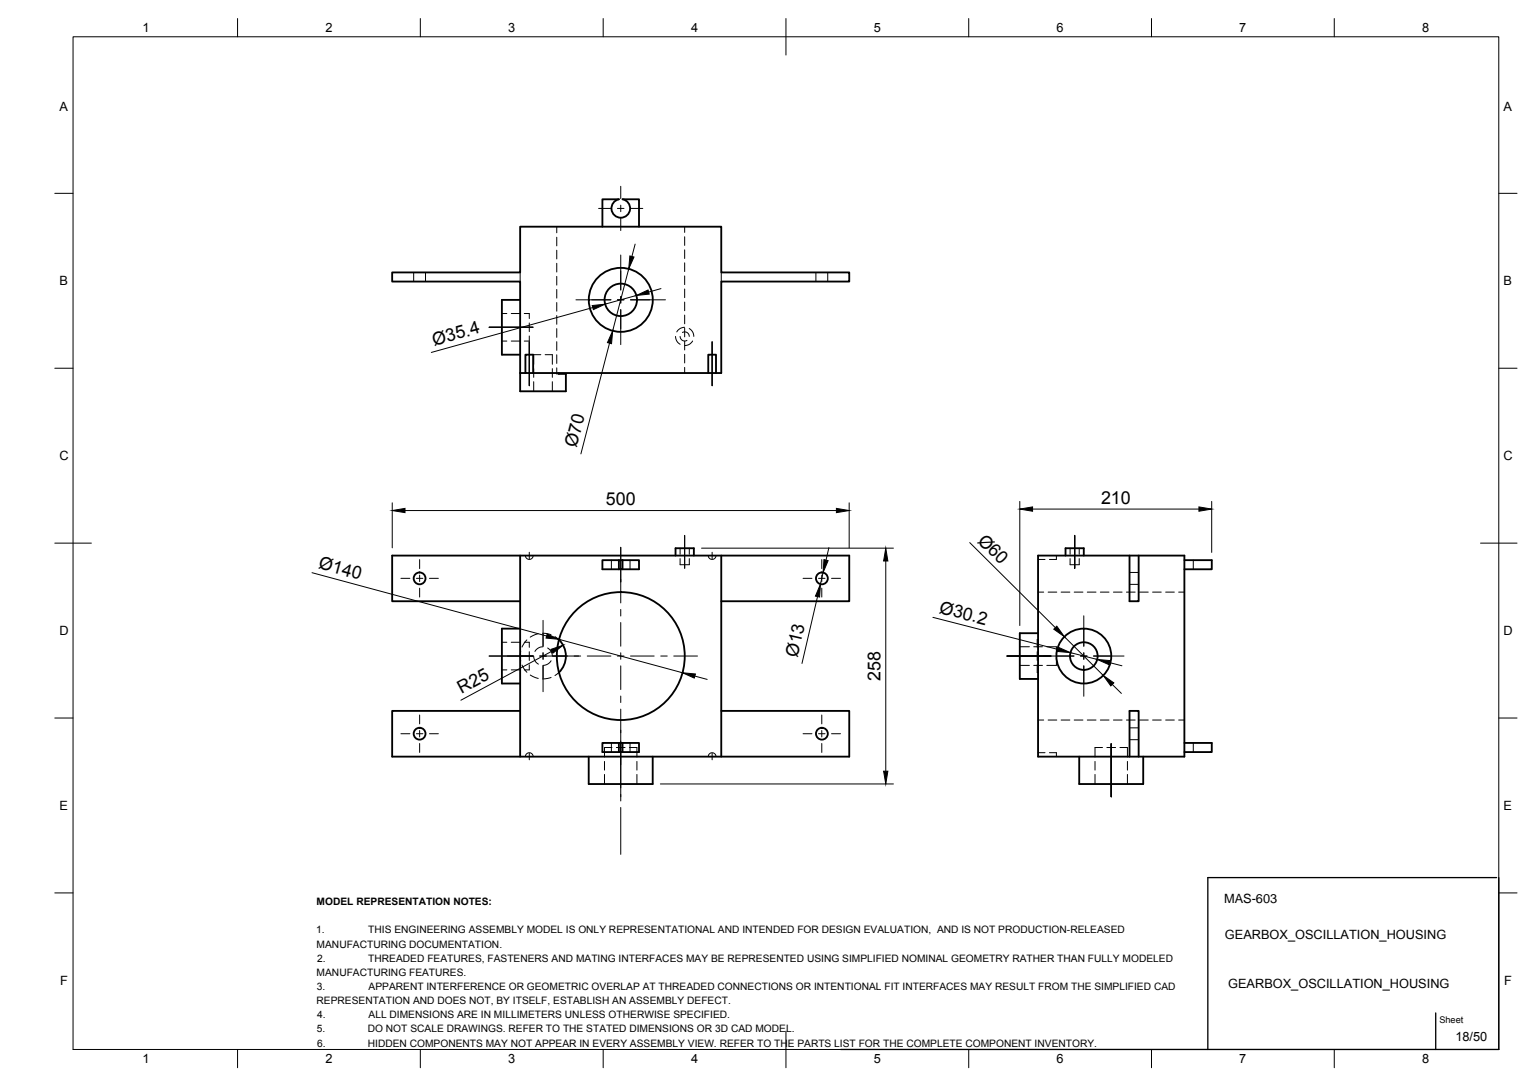
ISO-10303-21;
HEADER;
FILE_DESCRIPTION((''),'2;1');
FILE_NAME('GEARBOX_OSCILLATION_HOUSING.step','2026-10-01T22:06:14-07:00',(''),(''),'','','');
FILE_SCHEMA (('AUTOMOTIVE_DESIGN { 1 0 10303 214 3 1 1 }'));
ENDSEC;
DATA;
#10=MECHANICAL_DESIGN_GEOMETRIC_PRESENTATION_REPRESENTATION('',(#990),#50440);
#900=SHAPE_REPRESENTATION_RELATIONSHIP('SRR','None',#50632,#945) ;
#945=ADVANCED_BREP_SHAPE_REPRESENTATION('',(#1045),#50401) ;
#990=STYLED_ITEM('',(#50886),#1045) ;
#1045=MANIFOLD_SOLID_BREP('GEARBOX_OSCILLATION_HOUSING',#28657) ;
#1276=FACE_BOUND('',#4753,.T.) ;
#1277=FACE_BOUND('',#4757,.T.) ;
#1278=FACE_BOUND('',#4764,.T.) ;
#1279=FACE_BOUND('',#4785,.T.) ;
#1280=FACE_BOUND('',#4790,.T.) ;
#1281=FACE_BOUND('',#4795,.T.) ;
#1282=FACE_BOUND('',#4797,.T.) ;
#1283=FACE_BOUND('',#4799,.T.) ;
#1284=FACE_BOUND('',#4803,.T.) ;
#1285=FACE_BOUND('',#4805,.T.) ;
#1286=FACE_BOUND('',#4807,.T.) ;
#1287=FACE_BOUND('',#4811,.T.) ;
#1288=FACE_BOUND('',#4813,.T.) ;
#1289=FACE_BOUND('',#4817,.T.) ;
#1290=FACE_BOUND('',#4819,.T.) ;
#1291=FACE_BOUND('',#4824,.T.) ;
#1292=FACE_BOUND('',#4825,.T.) ;
#1293=FACE_BOUND('',#4826,.T.) ;
#1932=PLANE('',#30300) ;
#1933=PLANE('',#30301) ;
#1934=PLANE('',#30310) ;
#1935=PLANE('',#30313) ;
#1936=PLANE('',#30315) ;
#1937=PLANE('',#30318) ;
#1938=PLANE('',#30320) ;
#1939=PLANE('',#30326) ;
#1940=PLANE('',#30329) ;
#1941=PLANE('',#30336) ;
#1942=PLANE('',#30337) ;
#1943=PLANE('',#30338) ;
#1944=PLANE('',#30339) ;
#1945=PLANE('',#30340) ;
#1946=PLANE('',#30341) ;
#1947=PLANE('',#30342) ;
#1948=PLANE('',#30343) ;
#1949=PLANE('',#30344) ;
#1950=PLANE('',#30345) ;
#1951=PLANE('',#30346) ;
#1952=PLANE('',#30347) ;
#1953=PLANE('',#30348) ;
#1954=PLANE('',#30358) ;
#1955=PLANE('',#30359) ;
#1956=PLANE('',#30363) ;
#1957=PLANE('',#30367) ;
#1958=PLANE('',#30371) ;
#1959=PLANE('',#30374) ;
#1960=PLANE('',#30375) ;
#1961=PLANE('',#30376) ;
#1962=PLANE('',#30377) ;
#1963=PLANE('',#30378) ;
#1964=PLANE('',#30379) ;
#1965=PLANE('',#30380) ;
#1966=PLANE('',#30381) ;
#1967=PLANE('',#30382) ;
#1968=PLANE('',#30383) ;
#1969=PLANE('',#30384) ;
#1970=PLANE('',#30385) ;
#1971=PLANE('',#30386) ;
#1972=PLANE('',#30387) ;
#1973=PLANE('',#30388) ;
#1974=PLANE('',#30389) ;
#1975=PLANE('',#30390) ;
#1976=PLANE('',#30391) ;
#1977=PLANE('',#30392) ;
#1978=PLANE('',#30393) ;
#3025=FACE_OUTER_BOUND('',#4743,.T.) ;
#3026=FACE_OUTER_BOUND('',#4744,.T.) ;
#3027=FACE_OUTER_BOUND('',#4745,.T.) ;
#3028=FACE_OUTER_BOUND('',#4746,.T.) ;
#3029=FACE_OUTER_BOUND('',#4747,.T.) ;
#3030=FACE_OUTER_BOUND('',#4748,.T.) ;
#3031=FACE_OUTER_BOUND('',#4749,.T.) ;
#3032=FACE_OUTER_BOUND('',#4750,.T.) ;
#3033=FACE_OUTER_BOUND('',#4751,.T.) ;
#3034=FACE_OUTER_BOUND('',#4752,.T.) ;
#3035=FACE_OUTER_BOUND('',#4754,.T.) ;
#3036=FACE_OUTER_BOUND('',#4755,.T.) ;
#3037=FACE_OUTER_BOUND('',#4756,.T.) ;
#3038=FACE_OUTER_BOUND('',#4758,.T.) ;
#3039=FACE_OUTER_BOUND('',#4759,.T.) ;
#3040=FACE_OUTER_BOUND('',#4760,.T.) ;
#3041=FACE_OUTER_BOUND('',#4761,.T.) ;
#3042=FACE_OUTER_BOUND('',#4762,.T.) ;
#3043=FACE_OUTER_BOUND('',#4763,.T.) ;
#3044=FACE_OUTER_BOUND('',#4765,.T.) ;
#3045=FACE_OUTER_BOUND('',#4766,.T.) ;
#3046=FACE_OUTER_BOUND('',#4767,.T.) ;
#3047=FACE_OUTER_BOUND('',#4768,.T.) ;
#3048=FACE_OUTER_BOUND('',#4769,.T.) ;
#3049=FACE_OUTER_BOUND('',#4770,.T.) ;
#3050=FACE_OUTER_BOUND('',#4771,.T.) ;
#3051=FACE_OUTER_BOUND('',#4772,.T.) ;
#3052=FACE_OUTER_BOUND('',#4773,.T.) ;
#3053=FACE_OUTER_BOUND('',#4774,.T.) ;
#3054=FACE_OUTER_BOUND('',#4775,.T.) ;
#3055=FACE_OUTER_BOUND('',#4776,.T.) ;
#3056=FACE_OUTER_BOUND('',#4777,.T.) ;
#3057=FACE_OUTER_BOUND('',#4778,.T.) ;
#3058=FACE_OUTER_BOUND('',#4779,.T.) ;
#3059=FACE_OUTER_BOUND('',#4780,.T.) ;
#3060=FACE_OUTER_BOUND('',#4781,.T.) ;
#3061=FACE_OUTER_BOUND('',#4782,.T.) ;
#3062=FACE_OUTER_BOUND('',#4783,.T.) ;
#3063=FACE_OUTER_BOUND('',#4784,.T.) ;
#3064=FACE_OUTER_BOUND('',#4786,.T.) ;
#3065=FACE_OUTER_BOUND('',#4787,.T.) ;
#3066=FACE_OUTER_BOUND('',#4788,.T.) ;
#3067=FACE_OUTER_BOUND('',#4789,.T.) ;
#3068=FACE_OUTER_BOUND('',#4791,.T.) ;
#3069=FACE_OUTER_BOUND('',#4792,.T.) ;
#3070=FACE_OUTER_BOUND('',#4793,.T.) ;
#3071=FACE_OUTER_BOUND('',#4794,.T.) ;
#3072=FACE_OUTER_BOUND('',#4796,.T.) ;
#3073=FACE_OUTER_BOUND('',#4798,.T.) ;
#3074=FACE_OUTER_BOUND('',#4800,.T.) ;
#3075=FACE_OUTER_BOUND('',#4801,.T.) ;
#3076=FACE_OUTER_BOUND('',#4802,.T.) ;
#3077=FACE_OUTER_BOUND('',#4804,.T.) ;
#3078=FACE_OUTER_BOUND('',#4806,.T.) ;
#3079=FACE_OUTER_BOUND('',#4808,.T.) ;
#3080=FACE_OUTER_BOUND('',#4809,.T.) ;
#3081=FACE_OUTER_BOUND('',#4810,.T.) ;
#3082=FACE_OUTER_BOUND('',#4812,.T.) ;
#3083=FACE_OUTER_BOUND('',#4814,.T.) ;
#3084=FACE_OUTER_BOUND('',#4815,.T.) ;
#3085=FACE_OUTER_BOUND('',#4816,.T.) ;
#3086=FACE_OUTER_BOUND('',#4818,.T.) ;
#3087=FACE_OUTER_BOUND('',#4820,.T.) ;
#3088=FACE_OUTER_BOUND('',#4821,.T.) ;
#3089=FACE_OUTER_BOUND('',#4822,.T.) ;
#3090=FACE_OUTER_BOUND('',#4823,.T.) ;
#4743=EDGE_LOOP('',(#22155,#22156,#22157,#22158)) ;
#4744=EDGE_LOOP('',(#22159,#22160,#22161,#22162)) ;
#4745=EDGE_LOOP('',(#22163,#22164,#22165,#22166)) ;
#4746=EDGE_LOOP('',(#22167,#22168,#22169,#22170)) ;
#4747=EDGE_LOOP('',(#22171,#22172,#22173,#22174)) ;
#4748=EDGE_LOOP('',(#22175,#22176)) ;
#4749=EDGE_LOOP('',(#22177,#22178,#22179,#22180,#22181,#22182,#22183,#22184,
#22185,#22186,#22187,#22188,#22189,#22190,#22191,#22192,#22193,#22194)) ;
#4750=EDGE_LOOP('',(#22195,#22196)) ;
#4751=EDGE_LOOP('',(#22197,#22198,#22199,#22200)) ;
#4752=EDGE_LOOP('',(#22201,#22202,#22203,#22204,#22205,#22206,#22207,#22208,
#22209,#22210,#22211,#22212,#22213,#22214,#22215,#22216,#22217,#22218,#22219,
#22220)) ;
#4753=EDGE_LOOP('',(#22221)) ;
#4754=EDGE_LOOP('',(#22222,#22223)) ;
#4755=EDGE_LOOP('',(#22224,#22225,#22226,#22227)) ;
#4756=EDGE_LOOP('',(#22228,#22229,#22230,#22231,#22232,#22233,#22234,#22235,
#22236,#22237,#22238,#22239,#22240,#22241,#22242,#22243,#22244,#22245,#22246,
#22247)) ;
#4757=EDGE_LOOP('',(#22248)) ;
#4758=EDGE_LOOP('',(#22249,#22250)) ;
#4759=EDGE_LOOP('',(#22251,#22252,#22253,#22254)) ;
#4760=EDGE_LOOP('',(#22255,#22256,#22257,#22258)) ;
#4761=EDGE_LOOP('',(#22259)) ;
#4762=EDGE_LOOP('',(#22260,#22261,#22262,#22263)) ;
#4763=EDGE_LOOP('',(#22264)) ;
#4764=EDGE_LOOP('',(#22265)) ;
#4765=EDGE_LOOP('',(#22266,#22267,#22268,#22269)) ;
#4766=EDGE_LOOP('',(#22270,#22271,#22272,#22273)) ;
#4767=EDGE_LOOP('',(#22274,#22275,#22276,#22277,#22278,#22279)) ;
#4768=EDGE_LOOP('',(#22280,#22281,#22282,#22283)) ;
#4769=EDGE_LOOP('',(#22284,#22285,#22286,#22287)) ;
#4770=EDGE_LOOP('',(#22288,#22289,#22290,#22291,#22292,#22293)) ;
#4771=EDGE_LOOP('',(#22294,#22295,#22296,#22297)) ;
#4772=EDGE_LOOP('',(#22298,#22299,#22300,#22301)) ;
#4773=EDGE_LOOP('',(#22302,#22303,#22304,#22305)) ;
#4774=EDGE_LOOP('',(#22306,#22307,#22308,#22309)) ;
#4775=EDGE_LOOP('',(#22310,#22311,#22312,#22313,#22314,#22315)) ;
#4776=EDGE_LOOP('',(#22316,#22317,#22318,#22319)) ;
#4777=EDGE_LOOP('',(#22320,#22321,#22322,#22323)) ;
#4778=EDGE_LOOP('',(#22324,#22325,#22326,#22327,#22328,#22329)) ;
#4779=EDGE_LOOP('',(#22330,#22331)) ;
#4780=EDGE_LOOP('',(#22332,#22333,#22334,#22335,#22336,#22337,#22338,#22339)) ;
#4781=EDGE_LOOP('',(#22340,#22341,#22342,#22343,#22344,#22345,#22346,#22347,
#22348)) ;
#4782=EDGE_LOOP('',(#22349,#22350,#22351,#22352)) ;
#4783=EDGE_LOOP('',(#22353)) ;
#4784=EDGE_LOOP('',(#22354)) ;
#4785=EDGE_LOOP('',(#22355)) ;
#4786=EDGE_LOOP('',(#22356,#22357,#22358,#22359)) ;
#4787=EDGE_LOOP('',(#22360)) ;
#4788=EDGE_LOOP('',(#22361,#22362,#22363,#22364)) ;
#4789=EDGE_LOOP('',(#22365)) ;
#4790=EDGE_LOOP('',(#22366)) ;
#4791=EDGE_LOOP('',(#22367,#22368,#22369,#22370)) ;
#4792=EDGE_LOOP('',(#22371)) ;
#4793=EDGE_LOOP('',(#22372,#22373,#22374,#22375)) ;
#4794=EDGE_LOOP('',(#22376)) ;
#4795=EDGE_LOOP('',(#22377)) ;
#4796=EDGE_LOOP('',(#22378,#22379,#22380,#22381)) ;
#4797=EDGE_LOOP('',(#22382)) ;
#4798=EDGE_LOOP('',(#22383,#22384,#22385,#22386)) ;
#4799=EDGE_LOOP('',(#22387)) ;
#4800=EDGE_LOOP('',(#22388,#22389,#22390,#22391)) ;
#4801=EDGE_LOOP('',(#22392,#22393,#22394,#22395)) ;
#4802=EDGE_LOOP('',(#22396,#22397,#22398,#22399,#22400,#22401,#22402,#22403,
#22404,#22405,#22406,#22407,#22408)) ;
#4803=EDGE_LOOP('',(#22409)) ;
#4804=EDGE_LOOP('',(#22410,#22411,#22412,#22413)) ;
#4805=EDGE_LOOP('',(#22414)) ;
#4806=EDGE_LOOP('',(#22415,#22416,#22417,#22418)) ;
#4807=EDGE_LOOP('',(#22419)) ;
#4808=EDGE_LOOP('',(#22420,#22421,#22422,#22423)) ;
#4809=EDGE_LOOP('',(#22424,#22425,#22426,#22427)) ;
#4810=EDGE_LOOP('',(#22428,#22429,#22430,#22431)) ;
#4811=EDGE_LOOP('',(#22432)) ;
#4812=EDGE_LOOP('',(#22433,#22434,#22435,#22436)) ;
#4813=EDGE_LOOP('',(#22437)) ;
#4814=EDGE_LOOP('',(#22438,#22439,#22440,#22441)) ;
#4815=EDGE_LOOP('',(#22442,#22443,#22444,#22445)) ;
#4816=EDGE_LOOP('',(#22446,#22447,#22448,#22449)) ;
#4817=EDGE_LOOP('',(#22450)) ;
#4818=EDGE_LOOP('',(#22451,#22452,#22453,#22454)) ;
#4819=EDGE_LOOP('',(#22455)) ;
#4820=EDGE_LOOP('',(#22456,#22457,#22458,#22459)) ;
#4821=EDGE_LOOP('',(#22460,#22461,#22462,#22463)) ;
#4822=EDGE_LOOP('',(#22464,#22465,#22466,#22467,#22468,#22469,#22470,#22471,
#22472,#22473,#22474,#22475)) ;
#4823=EDGE_LOOP('',(#22476,#22477,#22478,#22479)) ;
#4824=EDGE_LOOP('',(#22480,#22481,#22482,#22483)) ;
#4825=EDGE_LOOP('',(#22484,#22485,#22486,#22487)) ;
#4826=EDGE_LOOP('',(#22488)) ;
#7141=LINE('',#45071,#9613) ;
#7142=LINE('',#45077,#9614) ;
#7143=LINE('',#45083,#9615) ;
#7144=LINE('',#45089,#9616) ;
#7145=LINE('',#45094,#9617) ;
#7146=LINE('',#45098,#9618) ;
#7147=LINE('',#45101,#9619) ;
#7148=LINE('',#45104,#9620) ;
#7149=LINE('',#45106,#9621) ;
#7150=LINE('',#45117,#9622) ;
#7151=LINE('',#45119,#9623) ;
#7152=LINE('',#45123,#9624) ;
#7153=LINE('',#45127,#9625) ;
#7154=LINE('',#45129,#9626) ;
#7155=LINE('',#45131,#9627) ;
#7156=LINE('',#45134,#9628) ;
#7157=LINE('',#45138,#9629) ;
#7158=LINE('',#45141,#9630) ;
#7159=LINE('',#45142,#9631) ;
#7160=LINE('',#45145,#9632) ;
#7161=LINE('',#45147,#9633) ;
#7162=LINE('',#45149,#9634) ;
#7163=LINE('',#45151,#9635) ;
#7164=LINE('',#45153,#9636) ;
#7165=LINE('',#45155,#9637) ;
#7166=LINE('',#45157,#9638) ;
#7167=LINE('',#45159,#9639) ;
#7168=LINE('',#45161,#9640) ;
#7169=LINE('',#45163,#9641) ;
#7170=LINE('',#45164,#9642) ;
#7171=LINE('',#45170,#9643) ;
#7172=LINE('',#45173,#9644) ;
#7173=LINE('',#45174,#9645) ;
#7174=LINE('',#45177,#9646) ;
#7175=LINE('',#45179,#9647) ;
#7176=LINE('',#45181,#9648) ;
#7177=LINE('',#45183,#9649) ;
#7178=LINE('',#45185,#9650) ;
#7179=LINE('',#45187,#9651) ;
#7180=LINE('',#45189,#9652) ;
#7181=LINE('',#45191,#9653) ;
#7182=LINE('',#45193,#9654) ;
#7183=LINE('',#45195,#9655) ;
#7184=LINE('',#45196,#9656) ;
#7185=LINE('',#45198,#9657) ;
#7186=LINE('',#45200,#9658) ;
#7187=LINE('',#45201,#9659) ;
#7188=LINE('',#45211,#9660) ;
#7189=LINE('',#45217,#9661) ;
#7190=LINE('',#45222,#9662) ;
#7191=LINE('',#45226,#9663) ;
#7192=LINE('',#45231,#9664) ;
#7193=LINE('',#45235,#9665) ;
#7194=LINE('',#45239,#9666) ;
#7195=LINE('',#45241,#9667) ;
#7196=LINE('',#45243,#9668) ;
#7197=LINE('',#45245,#9669) ;
#7198=LINE('',#45246,#9670) ;
#7199=LINE('',#45249,#9671) ;
#7200=LINE('',#45250,#9672) ;
#7201=LINE('',#45253,#9673) ;
#7202=LINE('',#45254,#9674) ;
#7203=LINE('',#45257,#9675) ;
#7204=LINE('',#45259,#9676) ;
#7205=LINE('',#45261,#9677) ;
#7206=LINE('',#45263,#9678) ;
#7207=LINE('',#45264,#9679) ;
#7208=LINE('',#45267,#9680) ;
#7209=LINE('',#45268,#9681) ;
#7210=LINE('',#45271,#9682) ;
#7211=LINE('',#45272,#9683) ;
#7212=LINE('',#45275,#9684) ;
#7213=LINE('',#45276,#9685) ;
#7214=LINE('',#45279,#9686) ;
#7215=LINE('',#45280,#9687) ;
#7216=LINE('',#45282,#9688) ;
#7217=LINE('',#45285,#9689) ;
#7218=LINE('',#45286,#9690) ;
#7219=LINE('',#45289,#9691) ;
#7220=LINE('',#45290,#9692) ;
#7221=LINE('',#45292,#9693) ;
#7222=LINE('',#45301,#9694) ;
#7223=LINE('',#45302,#9695) ;
#7224=LINE('',#45303,#9696) ;
#7225=LINE('',#45307,#9697) ;
#7226=LINE('',#45312,#9698) ;
#7227=LINE('',#45320,#9699) ;
#7228=LINE('',#45327,#9700) ;
#7229=LINE('',#45334,#9701) ;
#7230=LINE('',#45339,#9702) ;
#7231=LINE('',#45345,#9703) ;
#7232=LINE('',#45346,#9704) ;
#7233=LINE('',#45347,#9705) ;
#7234=LINE('',#45351,#9706) ;
#7235=LINE('',#45352,#9707) ;
#7236=LINE('',#45353,#9708) ;
#7237=LINE('',#45355,#9709) ;
#7238=LINE('',#45357,#9710) ;
#7239=LINE('',#45359,#9711) ;
#7240=LINE('',#45361,#9712) ;
#7241=LINE('',#45363,#9713) ;
#7242=LINE('',#45364,#9714) ;
#7243=LINE('',#45368,#9715) ;
#7244=LINE('',#45369,#9716) ;
#7245=LINE('',#45370,#9717) ;
#7246=LINE('',#45374,#9718) ;
#7247=LINE('',#45375,#9719) ;
#7248=LINE('',#45376,#9720) ;
#7249=LINE('',#45378,#9721) ;
#7250=LINE('',#45380,#9722) ;
#7251=LINE('',#45383,#9723) ;
#7252=LINE('',#45384,#9724) ;
#7253=LINE('',#45387,#9725) ;
#7254=LINE('',#45388,#9726) ;
#7255=LINE('',#45390,#9727) ;
#7256=LINE('',#45394,#9728) ;
#7257=LINE('',#45396,#9729) ;
#7258=LINE('',#45397,#9730) ;
#7259=LINE('',#45400,#9731) ;
#7260=LINE('',#45402,#9732) ;
#7261=LINE('',#45403,#9733) ;
#7262=LINE('',#45405,#9734) ;
#7263=LINE('',#45406,#9735) ;
#7264=LINE('',#45409,#9736) ;
#9613=VECTOR('',#35940,0.65) ;
#9614=VECTOR('',#35947,0.65) ;
#9615=VECTOR('',#35954,0.65) ;
#9616=VECTOR('',#35961,0.65) ;
#9617=VECTOR('',#35966,1.) ;
#9618=VECTOR('',#35969,1.) ;
#9619=VECTOR('',#35974,1.) ;
#9620=VECTOR('',#35977,1.) ;
#9621=VECTOR('',#35978,1.) ;
#9622=VECTOR('',#35989,1.) ;
#9623=VECTOR('',#35990,1.) ;
#9624=VECTOR('',#35993,1.) ;
#9625=VECTOR('',#35996,1.) ;
#9626=VECTOR('',#35997,1.) ;
#9627=VECTOR('',#35998,1.) ;
#9628=VECTOR('',#36001,1.) ;
#9629=VECTOR('',#36004,1.) ;
#9630=VECTOR('',#36009,1.) ;
#9631=VECTOR('',#36010,1.) ;
#9632=VECTOR('',#36013,1.) ;
#9633=VECTOR('',#36014,1.) ;
#9634=VECTOR('',#36015,1.) ;
#9635=VECTOR('',#36016,1.) ;
#9636=VECTOR('',#36017,1.) ;
#9637=VECTOR('',#36018,1.) ;
#9638=VECTOR('',#36019,1.) ;
#9639=VECTOR('',#36020,1.) ;
#9640=VECTOR('',#36021,1.) ;
#9641=VECTOR('',#36022,1.) ;
#9642=VECTOR('',#36023,1.) ;
#9643=VECTOR('',#36028,1.) ;
#9644=VECTOR('',#36033,1.) ;
#9645=VECTOR('',#36034,1.) ;
#9646=VECTOR('',#36037,1.) ;
#9647=VECTOR('',#36038,1.) ;
#9648=VECTOR('',#36039,1.) ;
#9649=VECTOR('',#36040,1.) ;
#9650=VECTOR('',#36041,1.) ;
#9651=VECTOR('',#36042,1.) ;
#9652=VECTOR('',#36043,1.) ;
#9653=VECTOR('',#36044,1.) ;
#9654=VECTOR('',#36045,1.) ;
#9655=VECTOR('',#36046,1.) ;
#9656=VECTOR('',#36047,1.) ;
#9657=VECTOR('',#36048,1.) ;
#9658=VECTOR('',#36049,1.) ;
#9659=VECTOR('',#36050,1.) ;
#9660=VECTOR('',#36063,0.5) ;
#9661=VECTOR('',#36072,1.) ;
#9662=VECTOR('',#36077,1.) ;
#9663=VECTOR('',#36080,1.) ;
#9664=VECTOR('',#36085,1.) ;
#9665=VECTOR('',#36088,1.) ;
#9666=VECTOR('',#36093,1.) ;
#9667=VECTOR('',#36094,1.) ;
#9668=VECTOR('',#36095,1.) ;
#9669=VECTOR('',#36096,1.) ;
#9670=VECTOR('',#36097,1.) ;
#9671=VECTOR('',#36100,1.) ;
#9672=VECTOR('',#36101,1.) ;
#9673=VECTOR('',#36104,1.) ;
#9674=VECTOR('',#36105,1.) ;
#9675=VECTOR('',#36108,1.) ;
#9676=VECTOR('',#36109,1.) ;
#9677=VECTOR('',#36110,1.) ;
#9678=VECTOR('',#36111,1.) ;
#9679=VECTOR('',#36112,1.) ;
#9680=VECTOR('',#36115,1.) ;
#9681=VECTOR('',#36116,1.) ;
#9682=VECTOR('',#36119,1.) ;
#9683=VECTOR('',#36120,1.) ;
#9684=VECTOR('',#36123,1.) ;
#9685=VECTOR('',#36124,1.) ;
#9686=VECTOR('',#36127,1.) ;
#9687=VECTOR('',#36128,1.) ;
#9688=VECTOR('',#36131,1.) ;
#9689=VECTOR('',#36134,1.) ;
#9690=VECTOR('',#36135,1.) ;
#9691=VECTOR('',#36138,1.) ;
#9692=VECTOR('',#36139,1.) ;
#9693=VECTOR('',#36142,1.) ;
#9694=VECTOR('',#36153,7.) ;
#9695=VECTOR('',#36154,1.) ;
#9696=VECTOR('',#36155,1.) ;
#9697=VECTOR('',#36160,2.5) ;
#9698=VECTOR('',#36165,1.02) ;
#9699=VECTOR('',#36176,1.51) ;
#9700=VECTOR('',#36185,3.) ;
#9701=VECTOR('',#36194,1.77) ;
#9702=VECTOR('',#36201,3.5) ;
#9703=VECTOR('',#36208,1.) ;
#9704=VECTOR('',#36209,1.) ;
#9705=VECTOR('',#36210,1.) ;
#9706=VECTOR('',#36213,1.) ;
#9707=VECTOR('',#36214,1.) ;
#9708=VECTOR('',#36215,1.) ;
#9709=VECTOR('',#36218,1.) ;
#9710=VECTOR('',#36221,1.) ;
#9711=VECTOR('',#36224,1.) ;
#9712=VECTOR('',#36225,1.) ;
#9713=VECTOR('',#36226,1.) ;
#9714=VECTOR('',#36227,1.) ;
#9715=VECTOR('',#36230,1.) ;
#9716=VECTOR('',#36231,1.) ;
#9717=VECTOR('',#36232,1.) ;
#9718=VECTOR('',#36235,1.) ;
#9719=VECTOR('',#36236,1.) ;
#9720=VECTOR('',#36237,1.) ;
#9721=VECTOR('',#36240,1.) ;
#9722=VECTOR('',#36243,1.) ;
#9723=VECTOR('',#36246,1.) ;
#9724=VECTOR('',#36247,1.) ;
#9725=VECTOR('',#36250,1.) ;
#9726=VECTOR('',#36251,1.) ;
#9727=VECTOR('',#36254,1.) ;
#9728=VECTOR('',#36259,1.) ;
#9729=VECTOR('',#36260,1.) ;
#9730=VECTOR('',#36261,1.) ;
#9731=VECTOR('',#36264,1.) ;
#9732=VECTOR('',#36265,1.) ;
#9733=VECTOR('',#36266,1.) ;
#9734=VECTOR('',#36269,1.) ;
#9735=VECTOR('',#36270,1.) ;
#9736=VECTOR('',#36275,1.) ;
#11006=CIRCLE('',#30286,0.65) ;
#11007=CIRCLE('',#30287,0.65) ;
#11008=CIRCLE('',#30289,0.65) ;
#11009=CIRCLE('',#30290,0.65) ;
#11010=CIRCLE('',#30292,0.65) ;
#11011=CIRCLE('',#30293,0.65) ;
#11012=CIRCLE('',#30295,0.65) ;
#11013=CIRCLE('',#30296,0.65) ;
#11014=CIRCLE('',#30298,0.425) ;
#11015=CIRCLE('',#30299,0.425) ;
#11016=CIRCLE('',#30302,2.5) ;
#11017=CIRCLE('',#30303,2.5) ;
#11018=CIRCLE('',#30304,7.) ;
#11019=CIRCLE('',#30305,7.) ;
#11020=CIRCLE('',#30306,2.5) ;
#11021=CIRCLE('',#30307,0.425) ;
#11022=CIRCLE('',#30308,0.425) ;
#11023=CIRCLE('',#30309,0.425) ;
#11024=CIRCLE('',#30311,0.425) ;
#11025=CIRCLE('',#30314,3.5) ;
#11026=CIRCLE('',#30316,0.425) ;
#11027=CIRCLE('',#30319,1.) ;
#11028=CIRCLE('',#30321,0.425) ;
#11029=CIRCLE('',#30324,0.5) ;
#11030=CIRCLE('',#30325,0.5) ;
#11031=CIRCLE('',#30328,1.) ;
#11032=CIRCLE('',#30331,1.02) ;
#11033=CIRCLE('',#30332,1.02) ;
#11034=CIRCLE('',#30334,1.02) ;
#11035=CIRCLE('',#30335,1.02) ;
#11036=CIRCLE('',#30349,2.5) ;
#11037=CIRCLE('',#30350,7.) ;
#11038=CIRCLE('',#30352,7.) ;
#11039=CIRCLE('',#30354,2.5) ;
#11040=CIRCLE('',#30356,1.02) ;
#11041=CIRCLE('',#30357,1.02) ;
#11042=CIRCLE('',#30361,1.51) ;
#11043=CIRCLE('',#30362,1.51) ;
#11044=CIRCLE('',#30365,3.) ;
#11045=CIRCLE('',#30366,3.) ;
#11046=CIRCLE('',#30369,1.77) ;
#11047=CIRCLE('',#30370,1.77) ;
#11048=CIRCLE('',#30373,3.5) ;
#13036=VERTEX_POINT('',#45068) ;
#13037=VERTEX_POINT('',#45070) ;
#13038=VERTEX_POINT('',#45074) ;
#13039=VERTEX_POINT('',#45076) ;
#13040=VERTEX_POINT('',#45080) ;
#13041=VERTEX_POINT('',#45082) ;
#13042=VERTEX_POINT('',#45086) ;
#13043=VERTEX_POINT('',#45088) ;
#13044=VERTEX_POINT('',#45092) ;
#13045=VERTEX_POINT('',#45093) ;
#13046=VERTEX_POINT('',#45095) ;
#13047=VERTEX_POINT('',#45097) ;
#13048=VERTEX_POINT('',#45103) ;
#13049=VERTEX_POINT('',#45105) ;
#13050=VERTEX_POINT('',#45107) ;
#13051=VERTEX_POINT('',#45109) ;
#13052=VERTEX_POINT('',#45111) ;
#13053=VERTEX_POINT('',#45113) ;
#13054=VERTEX_POINT('',#45116) ;
#13055=VERTEX_POINT('',#45118) ;
#13056=VERTEX_POINT('',#45120) ;
#13057=VERTEX_POINT('',#45122) ;
#13058=VERTEX_POINT('',#45124) ;
#13059=VERTEX_POINT('',#45126) ;
#13060=VERTEX_POINT('',#45128) ;
#13061=VERTEX_POINT('',#45130) ;
#13062=VERTEX_POINT('',#45132) ;
#13063=VERTEX_POINT('',#45136) ;
#13064=VERTEX_POINT('',#45137) ;
#13065=VERTEX_POINT('',#45144) ;
#13066=VERTEX_POINT('',#45146) ;
#13067=VERTEX_POINT('',#45148) ;
#13068=VERTEX_POINT('',#45150) ;
#13069=VERTEX_POINT('',#45152) ;
#13070=VERTEX_POINT('',#45154) ;
#13071=VERTEX_POINT('',#45156) ;
#13072=VERTEX_POINT('',#45158) ;
#13073=VERTEX_POINT('',#45160) ;
#13074=VERTEX_POINT('',#45162) ;
#13075=VERTEX_POINT('',#45165) ;
#13076=VERTEX_POINT('',#45168) ;
#13077=VERTEX_POINT('',#45169) ;
#13078=VERTEX_POINT('',#45176) ;
#13079=VERTEX_POINT('',#45178) ;
#13080=VERTEX_POINT('',#45180) ;
#13081=VERTEX_POINT('',#45182) ;
#13082=VERTEX_POINT('',#45184) ;
#13083=VERTEX_POINT('',#45186) ;
#13084=VERTEX_POINT('',#45188) ;
#13085=VERTEX_POINT('',#45190) ;
#13086=VERTEX_POINT('',#45192) ;
#13087=VERTEX_POINT('',#45194) ;
#13088=VERTEX_POINT('',#45197) ;
#13089=VERTEX_POINT('',#45199) ;
#13090=VERTEX_POINT('',#45202) ;
#13091=VERTEX_POINT('',#45208) ;
#13092=VERTEX_POINT('',#45210) ;
#13093=VERTEX_POINT('',#45215) ;
#13094=VERTEX_POINT('',#45220) ;
#13095=VERTEX_POINT('',#45221) ;
#13096=VERTEX_POINT('',#45223) ;
#13097=VERTEX_POINT('',#45225) ;
#13098=VERTEX_POINT('',#45229) ;
#13099=VERTEX_POINT('',#45230) ;
#13100=VERTEX_POINT('',#45232) ;
#13101=VERTEX_POINT('',#45234) ;
#13102=VERTEX_POINT('',#45238) ;
#13103=VERTEX_POINT('',#45240) ;
#13104=VERTEX_POINT('',#45242) ;
#13105=VERTEX_POINT('',#45244) ;
#13106=VERTEX_POINT('',#45248) ;
#13107=VERTEX_POINT('',#45252) ;
#13108=VERTEX_POINT('',#45256) ;
#13109=VERTEX_POINT('',#45258) ;
#13110=VERTEX_POINT('',#45260) ;
#13111=VERTEX_POINT('',#45262) ;
#13112=VERTEX_POINT('',#45266) ;
#13113=VERTEX_POINT('',#45270) ;
#13114=VERTEX_POINT('',#45274) ;
#13115=VERTEX_POINT('',#45278) ;
#13116=VERTEX_POINT('',#45284) ;
#13117=VERTEX_POINT('',#45288) ;
#13118=VERTEX_POINT('',#45294) ;
#13119=VERTEX_POINT('',#45295) ;
#13120=VERTEX_POINT('',#45299) ;
#13121=VERTEX_POINT('',#45305) ;
#13122=VERTEX_POINT('',#45309) ;
#13123=VERTEX_POINT('',#45311) ;
#13124=VERTEX_POINT('',#45317) ;
#13125=VERTEX_POINT('',#45319) ;
#13126=VERTEX_POINT('',#45324) ;
#13127=VERTEX_POINT('',#45326) ;
#13128=VERTEX_POINT('',#45331) ;
#13129=VERTEX_POINT('',#45333) ;
#13130=VERTEX_POINT('',#45338) ;
#13131=VERTEX_POINT('',#45343) ;
#13132=VERTEX_POINT('',#45344) ;
#13133=VERTEX_POINT('',#45349) ;
#13134=VERTEX_POINT('',#45350) ;
#13135=VERTEX_POINT('',#45360) ;
#13136=VERTEX_POINT('',#45362) ;
#13137=VERTEX_POINT('',#45366) ;
#13138=VERTEX_POINT('',#45367) ;
#13139=VERTEX_POINT('',#45372) ;
#13140=VERTEX_POINT('',#45373) ;
#13141=VERTEX_POINT('',#45382) ;
#13142=VERTEX_POINT('',#45386) ;
#13143=VERTEX_POINT('',#45393) ;
#13144=VERTEX_POINT('',#45395) ;
#13145=VERTEX_POINT('',#45399) ;
#13146=VERTEX_POINT('',#45401) ;
#16343=EDGE_CURVE('',#13036,#13036,#11006,.T.) ;
#16344=EDGE_CURVE('',#13036,#13037,#7141,.T.) ;
#16345=EDGE_CURVE('',#13037,#13037,#11007,.T.) ;
#16346=EDGE_CURVE('',#13038,#13038,#11008,.T.) ;
#16347=EDGE_CURVE('',#13038,#13039,#7142,.T.) ;
#16348=EDGE_CURVE('',#13039,#13039,#11009,.T.) ;
#16349=EDGE_CURVE('',#13040,#13040,#11010,.T.) ;
#16350=EDGE_CURVE('',#13040,#13041,#7143,.T.) ;
#16351=EDGE_CURVE('',#13041,#13041,#11011,.T.) ;
#16352=EDGE_CURVE('',#13042,#13042,#11012,.T.) ;
#16353=EDGE_CURVE('',#13042,#13043,#7144,.T.) ;
#16354=EDGE_CURVE('',#13043,#13043,#11013,.T.) ;
#16355=EDGE_CURVE('',#13044,#13045,#7145,.T.) ;
#16356=EDGE_CURVE('',#13044,#13046,#11014,.T.) ;
#16357=EDGE_CURVE('',#13047,#13046,#7146,.T.) ;
#16358=EDGE_CURVE('',#13045,#13047,#11015,.T.) ;
#16359=EDGE_CURVE('',#13046,#13044,#7147,.T.) ;
#16360=EDGE_CURVE('',#13047,#13048,#7148,.T.) ;
#16361=EDGE_CURVE('',#13048,#13049,#7149,.T.) ;
#16362=EDGE_CURVE('',#13049,#13050,#11016,.T.) ;
#16363=EDGE_CURVE('',#13050,#13051,#11017,.T.) ;
#16364=EDGE_CURVE('',#13051,#13052,#11018,.T.) ;
#16365=EDGE_CURVE('',#13052,#13053,#11019,.T.) ;
#16366=EDGE_CURVE('',#13053,#13049,#11020,.T.) ;
#16367=EDGE_CURVE('',#13049,#13054,#7150,.T.) ;
#16368=EDGE_CURVE('',#13054,#13055,#7151,.T.) ;
#16369=EDGE_CURVE('',#13055,#13056,#11021,.T.) ;
#16370=EDGE_CURVE('',#13056,#13057,#7152,.T.) ;
#16371=EDGE_CURVE('',#13057,#13058,#11022,.T.) ;
#16372=EDGE_CURVE('',#13058,#13059,#7153,.T.) ;
#16373=EDGE_CURVE('',#13059,#13060,#7154,.T.) ;
#16374=EDGE_CURVE('',#13060,#13061,#7155,.T.) ;
#16375=EDGE_CURVE('',#13061,#13062,#11023,.T.) ;
#16376=EDGE_CURVE('',#13062,#13045,#7156,.T.) ;
#16377=EDGE_CURVE('',#13063,#13064,#7157,.T.) ;
#16378=EDGE_CURVE('',#13064,#13063,#11024,.T.) ;
#16379=EDGE_CURVE('',#13062,#13063,#7158,.T.) ;
#16380=EDGE_CURVE('',#13064,#13061,#7159,.T.) ;
#16381=EDGE_CURVE('',#13060,#13065,#7160,.T.) ;
#16382=EDGE_CURVE('',#13066,#13065,#7161,.T.) ;
#16383=EDGE_CURVE('',#13066,#13067,#7162,.T.) ;
#16384=EDGE_CURVE('',#13068,#13067,#7163,.T.) ;
#16385=EDGE_CURVE('',#13068,#13069,#7164,.T.) ;
#16386=EDGE_CURVE('',#13070,#13069,#7165,.T.) ;
#16387=EDGE_CURVE('',#13071,#13070,#7166,.T.) ;
#16388=EDGE_CURVE('',#13072,#13071,#7167,.T.) ;
#16389=EDGE_CURVE('',#13073,#13072,#7168,.T.) ;
#16390=EDGE_CURVE('',#13074,#13073,#7169,.T.) ;
#16391=EDGE_CURVE('',#13048,#13074,#7170,.T.) ;
#16392=EDGE_CURVE('',#13075,#13075,#11025,.T.) ;
#16393=EDGE_CURVE('',#13076,#13077,#7171,.T.) ;
#16394=EDGE_CURVE('',#13077,#13076,#11026,.T.) ;
#16395=EDGE_CURVE('',#13056,#13076,#7172,.T.) ;
#16396=EDGE_CURVE('',#13077,#13055,#7173,.T.) ;
#16397=EDGE_CURVE('',#13054,#13078,#7174,.T.) ;
#16398=EDGE_CURVE('',#13079,#13078,#7175,.T.) ;
#16399=EDGE_CURVE('',#13079,#13080,#7176,.T.) ;
#16400=EDGE_CURVE('',#13081,#13080,#7177,.T.) ;
#16401=EDGE_CURVE('',#13081,#13082,#7178,.T.) ;
#16402=EDGE_CURVE('',#13083,#13082,#7179,.T.) ;
#16403=EDGE_CURVE('',#13084,#13083,#7180,.T.) ;
#16404=EDGE_CURVE('',#13085,#13084,#7181,.T.) ;
#16405=EDGE_CURVE('',#13086,#13085,#7182,.T.) ;
#16406=EDGE_CURVE('',#13087,#13086,#7183,.T.) ;
#16407=EDGE_CURVE('',#13059,#13087,#7184,.T.) ;
#16408=EDGE_CURVE('',#13058,#13088,#7185,.T.) ;
#16409=EDGE_CURVE('',#13088,#13089,#7186,.T.) ;
#16410=EDGE_CURVE('',#13089,#13057,#7187,.T.) ;
#16411=EDGE_CURVE('',#13090,#13090,#11027,.T.) ;
#16412=EDGE_CURVE('',#13089,#13088,#11028,.T.) ;
#16413=EDGE_CURVE('',#13091,#13091,#11029,.T.) ;
#16414=EDGE_CURVE('',#13091,#13092,#7188,.T.) ;
#16415=EDGE_CURVE('',#13092,#13092,#11030,.T.) ;
#16416=EDGE_CURVE('',#13093,#13093,#11031,.T.) ;
#16417=EDGE_CURVE('',#13093,#13090,#7189,.T.) ;
#16418=EDGE_CURVE('',#13094,#13095,#7190,.T.) ;
#16419=EDGE_CURVE('',#13096,#13094,#11032,.T.) ;
#16420=EDGE_CURVE('',#13097,#13096,#7191,.T.) ;
#16421=EDGE_CURVE('',#13095,#13097,#11033,.T.) ;
#16422=EDGE_CURVE('',#13098,#13099,#7192,.T.) ;
#16423=EDGE_CURVE('',#13100,#13098,#11034,.T.) ;
#16424=EDGE_CURVE('',#13101,#13100,#7193,.T.) ;
#16425=EDGE_CURVE('',#13099,#13101,#11035,.T.) ;
#16426=EDGE_CURVE('',#13102,#13098,#7194,.T.) ;
#16427=EDGE_CURVE('',#13103,#13102,#7195,.T.) ;
#16428=EDGE_CURVE('',#13104,#13103,#7196,.T.) ;
#16429=EDGE_CURVE('',#13104,#13105,#7197,.T.) ;
#16430=EDGE_CURVE('',#13100,#13105,#7198,.T.) ;
#16431=EDGE_CURVE('',#13099,#13106,#7199,.T.) ;
#16432=EDGE_CURVE('',#13106,#13102,#7200,.T.) ;
#16433=EDGE_CURVE('',#13105,#13107,#7201,.T.) ;
#16434=EDGE_CURVE('',#13107,#13101,#7202,.T.) ;
#16435=EDGE_CURVE('',#13108,#13094,#7203,.T.) ;
#16436=EDGE_CURVE('',#13109,#13108,#7204,.T.) ;
#16437=EDGE_CURVE('',#13110,#13109,#7205,.T.) ;
#16438=EDGE_CURVE('',#13110,#13111,#7206,.T.) ;
#16439=EDGE_CURVE('',#13096,#13111,#7207,.T.) ;
#16440=EDGE_CURVE('',#13095,#13112,#7208,.T.) ;
#16441=EDGE_CURVE('',#13112,#13108,#7209,.T.) ;
#16442=EDGE_CURVE('',#13111,#13113,#7210,.T.) ;
#16443=EDGE_CURVE('',#13113,#13097,#7211,.T.) ;
#16444=EDGE_CURVE('',#13114,#13106,#7212,.T.) ;
#16445=EDGE_CURVE('',#13103,#13114,#7213,.T.) ;
#16446=EDGE_CURVE('',#13115,#13107,#7214,.T.) ;
#16447=EDGE_CURVE('',#13115,#13104,#7215,.T.) ;
#16448=EDGE_CURVE('',#13114,#13115,#7216,.T.) ;
#16449=EDGE_CURVE('',#13116,#13112,#7217,.T.) ;
#16450=EDGE_CURVE('',#13109,#13116,#7218,.T.) ;
#16451=EDGE_CURVE('',#13117,#13113,#7219,.T.) ;
#16452=EDGE_CURVE('',#13117,#13110,#7220,.T.) ;
#16453=EDGE_CURVE('',#13116,#13117,#7221,.T.) ;
#16454=EDGE_CURVE('',#13118,#13119,#11036,.T.) ;
#16455=EDGE_CURVE('',#13119,#13118,#11037,.T.) ;
#16456=EDGE_CURVE('',#13120,#13120,#11038,.T.) ;
#16457=EDGE_CURVE('',#13120,#13052,#7222,.T.) ;
#16458=EDGE_CURVE('',#13119,#13051,#7223,.T.) ;
#16459=EDGE_CURVE('',#13053,#13118,#7224,.T.) ;
#16460=EDGE_CURVE('',#13121,#13121,#11039,.T.) ;
#16461=EDGE_CURVE('',#13121,#13050,#7225,.T.) ;
#16462=EDGE_CURVE('',#13122,#13122,#11040,.T.) ;
#16463=EDGE_CURVE('',#13122,#13123,#7226,.T.) ;
#16464=EDGE_CURVE('',#13123,#13123,#11041,.T.) ;
#16465=EDGE_CURVE('',#13124,#13124,#11042,.T.) ;
#16466=EDGE_CURVE('',#13124,#13125,#7227,.T.) ;
#16467=EDGE_CURVE('',#13125,#13125,#11043,.T.) ;
#16468=EDGE_CURVE('',#13126,#13126,#11044,.T.) ;
#16469=EDGE_CURVE('',#13126,#13127,#7228,.T.) ;
#16470=EDGE_CURVE('',#13127,#13127,#11045,.T.) ;
#16471=EDGE_CURVE('',#13128,#13128,#11046,.T.) ;
#16472=EDGE_CURVE('',#13128,#13129,#7229,.T.) ;
#16473=EDGE_CURVE('',#13129,#13129,#11047,.T.) ;
#16474=EDGE_CURVE('',#13075,#13130,#7230,.T.) ;
#16475=EDGE_CURVE('',#13130,#13130,#11048,.T.) ;
#16476=EDGE_CURVE('',#13131,#13132,#7231,.T.) ;
#16477=EDGE_CURVE('',#13074,#13132,#7232,.T.) ;
#16478=EDGE_CURVE('',#13073,#13131,#7233,.T.) ;
#16479=EDGE_CURVE('',#13133,#13134,#7234,.T.) ;
#16480=EDGE_CURVE('',#13134,#13072,#7235,.T.) ;
#16481=EDGE_CURVE('',#13133,#13071,#7236,.T.) ;
#16482=EDGE_CURVE('',#13131,#13134,#7237,.T.) ;
#16483=EDGE_CURVE('',#13132,#13133,#7238,.T.) ;
#16484=EDGE_CURVE('',#13082,#13070,#7239,.T.) ;
#16485=EDGE_CURVE('',#13081,#13135,#7240,.T.) ;
#16486=EDGE_CURVE('',#13135,#13136,#7241,.T.) ;
#16487=EDGE_CURVE('',#13136,#13078,#7242,.T.) ;
#16488=EDGE_CURVE('',#13137,#13138,#7243,.T.) ;
#16489=EDGE_CURVE('',#13138,#13066,#7244,.T.) ;
#16490=EDGE_CURVE('',#13137,#13065,#7245,.T.) ;
#16491=EDGE_CURVE('',#13139,#13140,#7246,.T.) ;
#16492=EDGE_CURVE('',#13068,#13140,#7247,.T.) ;
#16493=EDGE_CURVE('',#13067,#13139,#7248,.T.) ;
#16494=EDGE_CURVE('',#13138,#13139,#7249,.T.) ;
#16495=EDGE_CURVE('',#13140,#13137,#7250,.T.) ;
#16496=EDGE_CURVE('',#13136,#13141,#7251,.T.) ;
#16497=EDGE_CURVE('',#13141,#13079,#7252,.T.) ;
#16498=EDGE_CURVE('',#13080,#13142,#7253,.T.) ;
#16499=EDGE_CURVE('',#13142,#13135,#7254,.T.) ;
#16500=EDGE_CURVE('',#13141,#13142,#7255,.T.) ;
#16501=EDGE_CURVE('',#13086,#13143,#7256,.T.) ;
#16502=EDGE_CURVE('',#13143,#13144,#7257,.T.) ;
#16503=EDGE_CURVE('',#13087,#13144,#7258,.T.) ;
#16504=EDGE_CURVE('',#13145,#13084,#7259,.T.) ;
#16505=EDGE_CURVE('',#13145,#13146,#7260,.T.) ;
#16506=EDGE_CURVE('',#13146,#13085,#7261,.T.) ;
#16507=EDGE_CURVE('',#13143,#13146,#7262,.T.) ;
#16508=EDGE_CURVE('',#13144,#13145,#7263,.T.) ;
#16509=EDGE_CURVE('',#13069,#13083,#7264,.T.) ;
#22155=ORIENTED_EDGE('',*,*,#16343,.F.) ;
#22156=ORIENTED_EDGE('',*,*,#16344,.T.) ;
#22157=ORIENTED_EDGE('',*,*,#16345,.F.) ;
#22158=ORIENTED_EDGE('',*,*,#16344,.F.) ;
#22159=ORIENTED_EDGE('',*,*,#16346,.F.) ;
#22160=ORIENTED_EDGE('',*,*,#16347,.T.) ;
#22161=ORIENTED_EDGE('',*,*,#16348,.F.) ;
#22162=ORIENTED_EDGE('',*,*,#16347,.F.) ;
#22163=ORIENTED_EDGE('',*,*,#16349,.F.) ;
#22164=ORIENTED_EDGE('',*,*,#16350,.T.) ;
#22165=ORIENTED_EDGE('',*,*,#16351,.F.) ;
#22166=ORIENTED_EDGE('',*,*,#16350,.F.) ;
#22167=ORIENTED_EDGE('',*,*,#16352,.F.) ;
#22168=ORIENTED_EDGE('',*,*,#16353,.T.) ;
#22169=ORIENTED_EDGE('',*,*,#16354,.F.) ;
#22170=ORIENTED_EDGE('',*,*,#16353,.F.) ;
#22171=ORIENTED_EDGE('',*,*,#16355,.F.) ;
#22172=ORIENTED_EDGE('',*,*,#16356,.T.) ;
#22173=ORIENTED_EDGE('',*,*,#16357,.F.) ;
#22174=ORIENTED_EDGE('',*,*,#16358,.F.) ;
#22175=ORIENTED_EDGE('',*,*,#16359,.F.) ;
#22176=ORIENTED_EDGE('',*,*,#16356,.F.) ;
#22177=ORIENTED_EDGE('',*,*,#16358,.T.) ;
#22178=ORIENTED_EDGE('',*,*,#16360,.T.) ;
#22179=ORIENTED_EDGE('',*,*,#16361,.T.) ;
#22180=ORIENTED_EDGE('',*,*,#16362,.T.) ;
#22181=ORIENTED_EDGE('',*,*,#16363,.T.) ;
#22182=ORIENTED_EDGE('',*,*,#16364,.T.) ;
#22183=ORIENTED_EDGE('',*,*,#16365,.T.) ;
#22184=ORIENTED_EDGE('',*,*,#16366,.T.) ;
#22185=ORIENTED_EDGE('',*,*,#16367,.T.) ;
#22186=ORIENTED_EDGE('',*,*,#16368,.T.) ;
#22187=ORIENTED_EDGE('',*,*,#16369,.T.) ;
#22188=ORIENTED_EDGE('',*,*,#16370,.T.) ;
#22189=ORIENTED_EDGE('',*,*,#16371,.T.) ;
#22190=ORIENTED_EDGE('',*,*,#16372,.T.) ;
#22191=ORIENTED_EDGE('',*,*,#16373,.T.) ;
#22192=ORIENTED_EDGE('',*,*,#16374,.T.) ;
#22193=ORIENTED_EDGE('',*,*,#16375,.T.) ;
#22194=ORIENTED_EDGE('',*,*,#16376,.T.) ;
#22195=ORIENTED_EDGE('',*,*,#16377,.F.) ;
#22196=ORIENTED_EDGE('',*,*,#16378,.F.) ;
#22197=ORIENTED_EDGE('',*,*,#16379,.F.) ;
#22198=ORIENTED_EDGE('',*,*,#16375,.F.) ;
#22199=ORIENTED_EDGE('',*,*,#16380,.F.) ;
#22200=ORIENTED_EDGE('',*,*,#16378,.T.) ;
#22201=ORIENTED_EDGE('',*,*,#16355,.T.) ;
#22202=ORIENTED_EDGE('',*,*,#16376,.F.) ;
#22203=ORIENTED_EDGE('',*,*,#16379,.T.) ;
#22204=ORIENTED_EDGE('',*,*,#16377,.T.) ;
#22205=ORIENTED_EDGE('',*,*,#16380,.T.) ;
#22206=ORIENTED_EDGE('',*,*,#16374,.F.) ;
#22207=ORIENTED_EDGE('',*,*,#16381,.T.) ;
#22208=ORIENTED_EDGE('',*,*,#16382,.F.) ;
#22209=ORIENTED_EDGE('',*,*,#16383,.T.) ;
#22210=ORIENTED_EDGE('',*,*,#16384,.F.) ;
#22211=ORIENTED_EDGE('',*,*,#16385,.T.) ;
#22212=ORIENTED_EDGE('',*,*,#16386,.F.) ;
#22213=ORIENTED_EDGE('',*,*,#16387,.F.) ;
#22214=ORIENTED_EDGE('',*,*,#16388,.F.) ;
#22215=ORIENTED_EDGE('',*,*,#16389,.F.) ;
#22216=ORIENTED_EDGE('',*,*,#16390,.F.) ;
#22217=ORIENTED_EDGE('',*,*,#16391,.F.) ;
#22218=ORIENTED_EDGE('',*,*,#16360,.F.) ;
#22219=ORIENTED_EDGE('',*,*,#16357,.T.) ;
#22220=ORIENTED_EDGE('',*,*,#16359,.T.) ;
#22221=ORIENTED_EDGE('',*,*,#16392,.T.) ;
#22222=ORIENTED_EDGE('',*,*,#16393,.F.) ;
#22223=ORIENTED_EDGE('',*,*,#16394,.F.) ;
#22224=ORIENTED_EDGE('',*,*,#16395,.F.) ;
#22225=ORIENTED_EDGE('',*,*,#16369,.F.) ;
#22226=ORIENTED_EDGE('',*,*,#16396,.F.) ;
#22227=ORIENTED_EDGE('',*,*,#16394,.T.) ;
#22228=ORIENTED_EDGE('',*,*,#16395,.T.) ;
#22229=ORIENTED_EDGE('',*,*,#16393,.T.) ;
#22230=ORIENTED_EDGE('',*,*,#16396,.T.) ;
#22231=ORIENTED_EDGE('',*,*,#16368,.F.) ;
#22232=ORIENTED_EDGE('',*,*,#16397,.T.) ;
#22233=ORIENTED_EDGE('',*,*,#16398,.F.) ;
#22234=ORIENTED_EDGE('',*,*,#16399,.T.) ;
#22235=ORIENTED_EDGE('',*,*,#16400,.F.) ;
#22236=ORIENTED_EDGE('',*,*,#16401,.T.) ;
#22237=ORIENTED_EDGE('',*,*,#16402,.F.) ;
#22238=ORIENTED_EDGE('',*,*,#16403,.F.) ;
#22239=ORIENTED_EDGE('',*,*,#16404,.F.) ;
#22240=ORIENTED_EDGE('',*,*,#16405,.F.) ;
#22241=ORIENTED_EDGE('',*,*,#16406,.F.) ;
#22242=ORIENTED_EDGE('',*,*,#16407,.F.) ;
#22243=ORIENTED_EDGE('',*,*,#16372,.F.) ;
#22244=ORIENTED_EDGE('',*,*,#16408,.T.) ;
#22245=ORIENTED_EDGE('',*,*,#16409,.T.) ;
#22246=ORIENTED_EDGE('',*,*,#16410,.T.) ;
#22247=ORIENTED_EDGE('',*,*,#16370,.F.) ;
#22248=ORIENTED_EDGE('',*,*,#16411,.T.) ;
#22249=ORIENTED_EDGE('',*,*,#16409,.F.) ;
#22250=ORIENTED_EDGE('',*,*,#16412,.F.) ;
#22251=ORIENTED_EDGE('',*,*,#16408,.F.) ;
#22252=ORIENTED_EDGE('',*,*,#16371,.F.) ;
#22253=ORIENTED_EDGE('',*,*,#16410,.F.) ;
#22254=ORIENTED_EDGE('',*,*,#16412,.T.) ;
#22255=ORIENTED_EDGE('',*,*,#16413,.T.) ;
#22256=ORIENTED_EDGE('',*,*,#16414,.T.) ;
#22257=ORIENTED_EDGE('',*,*,#16415,.F.) ;
#22258=ORIENTED_EDGE('',*,*,#16414,.F.) ;
#22259=ORIENTED_EDGE('',*,*,#16413,.F.) ;
#22260=ORIENTED_EDGE('',*,*,#16416,.F.) ;
#22261=ORIENTED_EDGE('',*,*,#16417,.T.) ;
#22262=ORIENTED_EDGE('',*,*,#16411,.F.) ;
#22263=ORIENTED_EDGE('',*,*,#16417,.F.) ;
#22264=ORIENTED_EDGE('',*,*,#16416,.T.) ;
#22265=ORIENTED_EDGE('',*,*,#16415,.T.) ;
#22266=ORIENTED_EDGE('',*,*,#16418,.F.) ;
#22267=ORIENTED_EDGE('',*,*,#16419,.F.) ;
#22268=ORIENTED_EDGE('',*,*,#16420,.F.) ;
#22269=ORIENTED_EDGE('',*,*,#16421,.F.) ;
#22270=ORIENTED_EDGE('',*,*,#16422,.F.) ;
#22271=ORIENTED_EDGE('',*,*,#16423,.F.) ;
#22272=ORIENTED_EDGE('',*,*,#16424,.F.) ;
#22273=ORIENTED_EDGE('',*,*,#16425,.F.) ;
#22274=ORIENTED_EDGE('',*,*,#16423,.T.) ;
#22275=ORIENTED_EDGE('',*,*,#16426,.F.) ;
#22276=ORIENTED_EDGE('',*,*,#16427,.F.) ;
#22277=ORIENTED_EDGE('',*,*,#16428,.F.) ;
#22278=ORIENTED_EDGE('',*,*,#16429,.T.) ;
#22279=ORIENTED_EDGE('',*,*,#16430,.F.) ;
#22280=ORIENTED_EDGE('',*,*,#16422,.T.) ;
#22281=ORIENTED_EDGE('',*,*,#16431,.T.) ;
#22282=ORIENTED_EDGE('',*,*,#16432,.T.) ;
#22283=ORIENTED_EDGE('',*,*,#16426,.T.) ;
#22284=ORIENTED_EDGE('',*,*,#16424,.T.) ;
#22285=ORIENTED_EDGE('',*,*,#16430,.T.) ;
#22286=ORIENTED_EDGE('',*,*,#16433,.T.) ;
#22287=ORIENTED_EDGE('',*,*,#16434,.T.) ;
#22288=ORIENTED_EDGE('',*,*,#16419,.T.) ;
#22289=ORIENTED_EDGE('',*,*,#16435,.F.) ;
#22290=ORIENTED_EDGE('',*,*,#16436,.F.) ;
#22291=ORIENTED_EDGE('',*,*,#16437,.F.) ;
#22292=ORIENTED_EDGE('',*,*,#16438,.T.) ;
#22293=ORIENTED_EDGE('',*,*,#16439,.F.) ;
#22294=ORIENTED_EDGE('',*,*,#16418,.T.) ;
#22295=ORIENTED_EDGE('',*,*,#16440,.T.) ;
#22296=ORIENTED_EDGE('',*,*,#16441,.T.) ;
#22297=ORIENTED_EDGE('',*,*,#16435,.T.) ;
#22298=ORIENTED_EDGE('',*,*,#16420,.T.) ;
#22299=ORIENTED_EDGE('',*,*,#16439,.T.) ;
#22300=ORIENTED_EDGE('',*,*,#16442,.T.) ;
#22301=ORIENTED_EDGE('',*,*,#16443,.T.) ;
#22302=ORIENTED_EDGE('',*,*,#16427,.T.) ;
#22303=ORIENTED_EDGE('',*,*,#16432,.F.) ;
#22304=ORIENTED_EDGE('',*,*,#16444,.F.) ;
#22305=ORIENTED_EDGE('',*,*,#16445,.F.) ;
#22306=ORIENTED_EDGE('',*,*,#16446,.T.) ;
#22307=ORIENTED_EDGE('',*,*,#16433,.F.) ;
#22308=ORIENTED_EDGE('',*,*,#16429,.F.) ;
#22309=ORIENTED_EDGE('',*,*,#16447,.F.) ;
#22310=ORIENTED_EDGE('',*,*,#16425,.T.) ;
#22311=ORIENTED_EDGE('',*,*,#16434,.F.) ;
#22312=ORIENTED_EDGE('',*,*,#16446,.F.) ;
#22313=ORIENTED_EDGE('',*,*,#16448,.F.) ;
#22314=ORIENTED_EDGE('',*,*,#16444,.T.) ;
#22315=ORIENTED_EDGE('',*,*,#16431,.F.) ;
#22316=ORIENTED_EDGE('',*,*,#16436,.T.) ;
#22317=ORIENTED_EDGE('',*,*,#16441,.F.) ;
#22318=ORIENTED_EDGE('',*,*,#16449,.F.) ;
#22319=ORIENTED_EDGE('',*,*,#16450,.F.) ;
#22320=ORIENTED_EDGE('',*,*,#16451,.T.) ;
#22321=ORIENTED_EDGE('',*,*,#16442,.F.) ;
#22322=ORIENTED_EDGE('',*,*,#16438,.F.) ;
#22323=ORIENTED_EDGE('',*,*,#16452,.F.) ;
#22324=ORIENTED_EDGE('',*,*,#16421,.T.) ;
#22325=ORIENTED_EDGE('',*,*,#16443,.F.) ;
#22326=ORIENTED_EDGE('',*,*,#16451,.F.) ;
#22327=ORIENTED_EDGE('',*,*,#16453,.F.) ;
#22328=ORIENTED_EDGE('',*,*,#16449,.T.) ;
#22329=ORIENTED_EDGE('',*,*,#16440,.F.) ;
#22330=ORIENTED_EDGE('',*,*,#16454,.F.) ;
#22331=ORIENTED_EDGE('',*,*,#16455,.F.) ;
#22332=ORIENTED_EDGE('',*,*,#16456,.F.) ;
#22333=ORIENTED_EDGE('',*,*,#16457,.T.) ;
#22334=ORIENTED_EDGE('',*,*,#16364,.F.) ;
#22335=ORIENTED_EDGE('',*,*,#16458,.F.) ;
#22336=ORIENTED_EDGE('',*,*,#16455,.T.) ;
#22337=ORIENTED_EDGE('',*,*,#16459,.F.) ;
#22338=ORIENTED_EDGE('',*,*,#16365,.F.) ;
#22339=ORIENTED_EDGE('',*,*,#16457,.F.) ;
#22340=ORIENTED_EDGE('',*,*,#16460,.F.) ;
#22341=ORIENTED_EDGE('',*,*,#16461,.T.) ;
#22342=ORIENTED_EDGE('',*,*,#16362,.F.) ;
#22343=ORIENTED_EDGE('',*,*,#16366,.F.) ;
#22344=ORIENTED_EDGE('',*,*,#16459,.T.) ;
#22345=ORIENTED_EDGE('',*,*,#16454,.T.) ;
#22346=ORIENTED_EDGE('',*,*,#16458,.T.) ;
#22347=ORIENTED_EDGE('',*,*,#16363,.F.) ;
#22348=ORIENTED_EDGE('',*,*,#16461,.F.) ;
#22349=ORIENTED_EDGE('',*,*,#16462,.T.) ;
#22350=ORIENTED_EDGE('',*,*,#16463,.T.) ;
#22351=ORIENTED_EDGE('',*,*,#16464,.F.) ;
#22352=ORIENTED_EDGE('',*,*,#16463,.F.) ;
#22353=ORIENTED_EDGE('',*,*,#16462,.F.) ;
#22354=ORIENTED_EDGE('',*,*,#16460,.T.) ;
#22355=ORIENTED_EDGE('',*,*,#16464,.T.) ;
#22356=ORIENTED_EDGE('',*,*,#16465,.F.) ;
#22357=ORIENTED_EDGE('',*,*,#16466,.T.) ;
#22358=ORIENTED_EDGE('',*,*,#16467,.T.) ;
#22359=ORIENTED_EDGE('',*,*,#16466,.F.) ;
#22360=ORIENTED_EDGE('',*,*,#16467,.F.) ;
#22361=ORIENTED_EDGE('',*,*,#16468,.F.) ;
#22362=ORIENTED_EDGE('',*,*,#16469,.T.) ;
#22363=ORIENTED_EDGE('',*,*,#16470,.F.) ;
#22364=ORIENTED_EDGE('',*,*,#16469,.F.) ;
#22365=ORIENTED_EDGE('',*,*,#16470,.T.) ;
#22366=ORIENTED_EDGE('',*,*,#16465,.T.) ;
#22367=ORIENTED_EDGE('',*,*,#16471,.F.) ;
#22368=ORIENTED_EDGE('',*,*,#16472,.T.) ;
#22369=ORIENTED_EDGE('',*,*,#16473,.T.) ;
#22370=ORIENTED_EDGE('',*,*,#16472,.F.) ;
#22371=ORIENTED_EDGE('',*,*,#16473,.F.) ;
#22372=ORIENTED_EDGE('',*,*,#16392,.F.) ;
#22373=ORIENTED_EDGE('',*,*,#16474,.T.) ;
#22374=ORIENTED_EDGE('',*,*,#16475,.F.) ;
#22375=ORIENTED_EDGE('',*,*,#16474,.F.) ;
#22376=ORIENTED_EDGE('',*,*,#16475,.T.) ;
#22377=ORIENTED_EDGE('',*,*,#16471,.T.) ;
#22378=ORIENTED_EDGE('',*,*,#16476,.T.) ;
#22379=ORIENTED_EDGE('',*,*,#16477,.F.) ;
#22380=ORIENTED_EDGE('',*,*,#16390,.T.) ;
#22381=ORIENTED_EDGE('',*,*,#16478,.T.) ;
#22382=ORIENTED_EDGE('',*,*,#16345,.T.) ;
#22383=ORIENTED_EDGE('',*,*,#16479,.T.) ;
#22384=ORIENTED_EDGE('',*,*,#16480,.T.) ;
#22385=ORIENTED_EDGE('',*,*,#16388,.T.) ;
#22386=ORIENTED_EDGE('',*,*,#16481,.F.) ;
#22387=ORIENTED_EDGE('',*,*,#16343,.T.) ;
#22388=ORIENTED_EDGE('',*,*,#16389,.T.) ;
#22389=ORIENTED_EDGE('',*,*,#16480,.F.) ;
#22390=ORIENTED_EDGE('',*,*,#16482,.F.) ;
#22391=ORIENTED_EDGE('',*,*,#16478,.F.) ;
#22392=ORIENTED_EDGE('',*,*,#16482,.T.) ;
#22393=ORIENTED_EDGE('',*,*,#16479,.F.) ;
#22394=ORIENTED_EDGE('',*,*,#16483,.F.) ;
#22395=ORIENTED_EDGE('',*,*,#16476,.F.) ;
#22396=ORIENTED_EDGE('',*,*,#16477,.T.) ;
#22397=ORIENTED_EDGE('',*,*,#16483,.T.) ;
#22398=ORIENTED_EDGE('',*,*,#16481,.T.) ;
#22399=ORIENTED_EDGE('',*,*,#16387,.T.) ;
#22400=ORIENTED_EDGE('',*,*,#16484,.F.) ;
#22401=ORIENTED_EDGE('',*,*,#16401,.F.) ;
#22402=ORIENTED_EDGE('',*,*,#16485,.T.) ;
#22403=ORIENTED_EDGE('',*,*,#16486,.T.) ;
#22404=ORIENTED_EDGE('',*,*,#16487,.T.) ;
#22405=ORIENTED_EDGE('',*,*,#16397,.F.) ;
#22406=ORIENTED_EDGE('',*,*,#16367,.F.) ;
#22407=ORIENTED_EDGE('',*,*,#16361,.F.) ;
#22408=ORIENTED_EDGE('',*,*,#16391,.T.) ;
#22409=ORIENTED_EDGE('',*,*,#16468,.T.) ;
#22410=ORIENTED_EDGE('',*,*,#16488,.T.) ;
#22411=ORIENTED_EDGE('',*,*,#16489,.T.) ;
#22412=ORIENTED_EDGE('',*,*,#16382,.T.) ;
#22413=ORIENTED_EDGE('',*,*,#16490,.F.) ;
#22414=ORIENTED_EDGE('',*,*,#16348,.T.) ;
#22415=ORIENTED_EDGE('',*,*,#16491,.T.) ;
#22416=ORIENTED_EDGE('',*,*,#16492,.F.) ;
#22417=ORIENTED_EDGE('',*,*,#16384,.T.) ;
#22418=ORIENTED_EDGE('',*,*,#16493,.T.) ;
#22419=ORIENTED_EDGE('',*,*,#16346,.T.) ;
#22420=ORIENTED_EDGE('',*,*,#16494,.T.) ;
#22421=ORIENTED_EDGE('',*,*,#16493,.F.) ;
#22422=ORIENTED_EDGE('',*,*,#16383,.F.) ;
#22423=ORIENTED_EDGE('',*,*,#16489,.F.) ;
#22424=ORIENTED_EDGE('',*,*,#16495,.F.) ;
#22425=ORIENTED_EDGE('',*,*,#16491,.F.) ;
#22426=ORIENTED_EDGE('',*,*,#16494,.F.) ;
#22427=ORIENTED_EDGE('',*,*,#16488,.F.) ;
#22428=ORIENTED_EDGE('',*,*,#16398,.T.) ;
#22429=ORIENTED_EDGE('',*,*,#16487,.F.) ;
#22430=ORIENTED_EDGE('',*,*,#16496,.T.) ;
#22431=ORIENTED_EDGE('',*,*,#16497,.T.) ;
#22432=ORIENTED_EDGE('',*,*,#16351,.T.) ;
#22433=ORIENTED_EDGE('',*,*,#16400,.T.) ;
#22434=ORIENTED_EDGE('',*,*,#16498,.T.) ;
#22435=ORIENTED_EDGE('',*,*,#16499,.T.) ;
#22436=ORIENTED_EDGE('',*,*,#16485,.F.) ;
#22437=ORIENTED_EDGE('',*,*,#16349,.T.) ;
#22438=ORIENTED_EDGE('',*,*,#16500,.T.) ;
#22439=ORIENTED_EDGE('',*,*,#16498,.F.) ;
#22440=ORIENTED_EDGE('',*,*,#16399,.F.) ;
#22441=ORIENTED_EDGE('',*,*,#16497,.F.) ;
#22442=ORIENTED_EDGE('',*,*,#16486,.F.) ;
#22443=ORIENTED_EDGE('',*,*,#16499,.F.) ;
#22444=ORIENTED_EDGE('',*,*,#16500,.F.) ;
#22445=ORIENTED_EDGE('',*,*,#16496,.F.) ;
#22446=ORIENTED_EDGE('',*,*,#16406,.T.) ;
#22447=ORIENTED_EDGE('',*,*,#16501,.T.) ;
#22448=ORIENTED_EDGE('',*,*,#16502,.T.) ;
#22449=ORIENTED_EDGE('',*,*,#16503,.F.) ;
#22450=ORIENTED_EDGE('',*,*,#16354,.T.) ;
#22451=ORIENTED_EDGE('',*,*,#16404,.T.) ;
#22452=ORIENTED_EDGE('',*,*,#16504,.F.) ;
#22453=ORIENTED_EDGE('',*,*,#16505,.T.) ;
#22454=ORIENTED_EDGE('',*,*,#16506,.T.) ;
#22455=ORIENTED_EDGE('',*,*,#16352,.T.) ;
#22456=ORIENTED_EDGE('',*,*,#16507,.T.) ;
#22457=ORIENTED_EDGE('',*,*,#16505,.F.) ;
#22458=ORIENTED_EDGE('',*,*,#16508,.F.) ;
#22459=ORIENTED_EDGE('',*,*,#16502,.F.) ;
#22460=ORIENTED_EDGE('',*,*,#16405,.T.) ;
#22461=ORIENTED_EDGE('',*,*,#16506,.F.) ;
#22462=ORIENTED_EDGE('',*,*,#16507,.F.) ;
#22463=ORIENTED_EDGE('',*,*,#16501,.F.) ;
#22464=ORIENTED_EDGE('',*,*,#16490,.T.) ;
#22465=ORIENTED_EDGE('',*,*,#16381,.F.) ;
#22466=ORIENTED_EDGE('',*,*,#16373,.F.) ;
#22467=ORIENTED_EDGE('',*,*,#16407,.T.) ;
#22468=ORIENTED_EDGE('',*,*,#16503,.T.) ;
#22469=ORIENTED_EDGE('',*,*,#16508,.T.) ;
#22470=ORIENTED_EDGE('',*,*,#16504,.T.) ;
#22471=ORIENTED_EDGE('',*,*,#16403,.T.) ;
#22472=ORIENTED_EDGE('',*,*,#16509,.F.) ;
#22473=ORIENTED_EDGE('',*,*,#16385,.F.) ;
#22474=ORIENTED_EDGE('',*,*,#16492,.T.) ;
#22475=ORIENTED_EDGE('',*,*,#16495,.T.) ;
#22476=ORIENTED_EDGE('',*,*,#16402,.T.) ;
#22477=ORIENTED_EDGE('',*,*,#16484,.T.) ;
#22478=ORIENTED_EDGE('',*,*,#16386,.T.) ;
#22479=ORIENTED_EDGE('',*,*,#16509,.T.) ;
#22480=ORIENTED_EDGE('',*,*,#16445,.T.) ;
#22481=ORIENTED_EDGE('',*,*,#16448,.T.) ;
#22482=ORIENTED_EDGE('',*,*,#16447,.T.) ;
#22483=ORIENTED_EDGE('',*,*,#16428,.T.) ;
#22484=ORIENTED_EDGE('',*,*,#16450,.T.) ;
#22485=ORIENTED_EDGE('',*,*,#16453,.T.) ;
#22486=ORIENTED_EDGE('',*,*,#16452,.T.) ;
#22487=ORIENTED_EDGE('',*,*,#16437,.T.) ;
#22488=ORIENTED_EDGE('',*,*,#16456,.T.) ;
#26782=CYLINDRICAL_SURFACE('',#30285,0.65) ;
#26783=CYLINDRICAL_SURFACE('',#30288,0.65) ;
#26784=CYLINDRICAL_SURFACE('',#30291,0.65) ;
#26785=CYLINDRICAL_SURFACE('',#30294,0.65) ;
#26786=CYLINDRICAL_SURFACE('',#30297,0.425) ;
#26787=CYLINDRICAL_SURFACE('',#30312,0.425) ;
#26788=CYLINDRICAL_SURFACE('',#30317,0.425) ;
#26789=CYLINDRICAL_SURFACE('',#30322,0.425) ;
#26790=CYLINDRICAL_SURFACE('',#30323,0.5) ;
#26791=CYLINDRICAL_SURFACE('',#30327,1.) ;
#26792=CYLINDRICAL_SURFACE('',#30330,1.02) ;
#26793=CYLINDRICAL_SURFACE('',#30333,1.02) ;
#26794=CYLINDRICAL_SURFACE('',#30351,7.) ;
#26795=CYLINDRICAL_SURFACE('',#30353,2.5) ;
#26796=CYLINDRICAL_SURFACE('',#30355,1.02) ;
#26797=CYLINDRICAL_SURFACE('',#30360,1.51) ;
#26798=CYLINDRICAL_SURFACE('',#30364,3.) ;
#26799=CYLINDRICAL_SURFACE('',#30368,1.77) ;
#26800=CYLINDRICAL_SURFACE('',#30372,3.5) ;
#27760=ADVANCED_FACE('',(#3025),#26782,.F.) ;
#27761=ADVANCED_FACE('',(#3026),#26783,.F.) ;
#27762=ADVANCED_FACE('',(#3027),#26784,.F.) ;
#27763=ADVANCED_FACE('',(#3028),#26785,.F.) ;
#27764=ADVANCED_FACE('',(#3029),#26786,.F.) ;
#27765=ADVANCED_FACE('',(#3030),#1932,.F.) ;
#27766=ADVANCED_FACE('',(#3031),#1933,.T.) ;
#27767=ADVANCED_FACE('',(#3032),#1934,.F.) ;
#27768=ADVANCED_FACE('',(#3033),#26787,.F.) ;
#27769=ADVANCED_FACE('',(#3034,#1276),#1935,.F.) ;
#27770=ADVANCED_FACE('',(#3035),#1936,.F.) ;
#27771=ADVANCED_FACE('',(#3036),#26788,.F.) ;
#27772=ADVANCED_FACE('',(#3037,#1277),#1937,.F.) ;
#27773=ADVANCED_FACE('',(#3038),#1938,.F.) ;
#27774=ADVANCED_FACE('',(#3039),#26789,.F.) ;
#27775=ADVANCED_FACE('',(#3040),#26790,.F.) ;
#27776=ADVANCED_FACE('',(#3041),#1939,.F.) ;
#27777=ADVANCED_FACE('',(#3042),#26791,.T.) ;
#27778=ADVANCED_FACE('',(#3043,#1278),#1940,.T.) ;
#27779=ADVANCED_FACE('',(#3044),#26792,.F.) ;
#27780=ADVANCED_FACE('',(#3045),#26793,.F.) ;
#27781=ADVANCED_FACE('',(#3046),#1941,.F.) ;
#27782=ADVANCED_FACE('',(#3047),#1942,.F.) ;
#27783=ADVANCED_FACE('',(#3048),#1943,.F.) ;
#27784=ADVANCED_FACE('',(#3049),#1944,.F.) ;
#27785=ADVANCED_FACE('',(#3050),#1945,.F.) ;
#27786=ADVANCED_FACE('',(#3051),#1946,.F.) ;
#27787=ADVANCED_FACE('',(#3052),#1947,.F.) ;
#27788=ADVANCED_FACE('',(#3053),#1948,.F.) ;
#27789=ADVANCED_FACE('',(#3054),#1949,.F.) ;
#27790=ADVANCED_FACE('',(#3055),#1950,.F.) ;
#27791=ADVANCED_FACE('',(#3056),#1951,.F.) ;
#27792=ADVANCED_FACE('',(#3057),#1952,.F.) ;
#27793=ADVANCED_FACE('',(#3058),#1953,.F.) ;
#27794=ADVANCED_FACE('',(#3059),#26794,.F.) ;
#27795=ADVANCED_FACE('',(#3060),#26795,.T.) ;
#27796=ADVANCED_FACE('',(#3061),#26796,.F.) ;
#27797=ADVANCED_FACE('',(#3062),#1954,.F.) ;
#27798=ADVANCED_FACE('',(#3063,#1279),#1955,.T.) ;
#27799=ADVANCED_FACE('',(#3064),#26797,.F.) ;
#27800=ADVANCED_FACE('',(#3065),#1956,.F.) ;
#27801=ADVANCED_FACE('',(#3066),#26798,.T.) ;
#27802=ADVANCED_FACE('',(#3067,#1280),#1957,.T.) ;
#27803=ADVANCED_FACE('',(#3068),#26799,.F.) ;
#27804=ADVANCED_FACE('',(#3069),#1958,.F.) ;
#27805=ADVANCED_FACE('',(#3070),#26800,.T.) ;
#27806=ADVANCED_FACE('',(#3071,#1281),#1959,.T.) ;
#27807=ADVANCED_FACE('',(#3072,#1282),#1960,.T.) ;
#27808=ADVANCED_FACE('',(#3073,#1283),#1961,.F.) ;
#27809=ADVANCED_FACE('',(#3074),#1962,.F.) ;
#27810=ADVANCED_FACE('',(#3075),#1963,.F.) ;
#27811=ADVANCED_FACE('',(#3076,#1284),#1964,.F.) ;
#27812=ADVANCED_FACE('',(#3077,#1285),#1965,.T.) ;
#27813=ADVANCED_FACE('',(#3078,#1286),#1966,.F.) ;
#27814=ADVANCED_FACE('',(#3079),#1967,.F.) ;
#27815=ADVANCED_FACE('',(#3080),#1968,.F.) ;
#27816=ADVANCED_FACE('',(#3081,#1287),#1969,.T.) ;
#27817=ADVANCED_FACE('',(#3082,#1288),#1970,.F.) ;
#27818=ADVANCED_FACE('',(#3083),#1971,.F.) ;
#27819=ADVANCED_FACE('',(#3084),#1972,.F.) ;
#27820=ADVANCED_FACE('',(#3085,#1289),#1973,.T.) ;
#27821=ADVANCED_FACE('',(#3086,#1290),#1974,.F.) ;
#27822=ADVANCED_FACE('',(#3087),#1975,.F.) ;
#27823=ADVANCED_FACE('',(#3088),#1976,.F.) ;
#27824=ADVANCED_FACE('',(#3089),#1977,.F.) ;
#27825=ADVANCED_FACE('',(#3090,#1291,#1292,#1293),#1978,.F.) ;
#28657=CLOSED_SHELL('',(#27760,#27761,#27762,#27763,#27764,#27765,#27766,
#27767,#27768,#27769,#27770,#27771,#27772,#27773,#27774,#27775,#27776,#27777,
#27778,#27779,#27780,#27781,#27782,#27783,#27784,#27785,#27786,#27787,#27788,
#27789,#27790,#27791,#27792,#27793,#27794,#27795,#27796,#27797,#27798,#27799,
#27800,#27801,#27802,#27803,#27804,#27805,#27806,#27807,#27808,#27809,#27810,
#27811,#27812,#27813,#27814,#27815,#27816,#27817,#27818,#27819,#27820,#27821,
#27822,#27823,#27824,#27825)) ;
#30284=AXIS2_PLACEMENT_3D('',#45066,#35934,#35935) ;
#30285=AXIS2_PLACEMENT_3D('',#45067,#35936,#35937) ;
#30286=AXIS2_PLACEMENT_3D('',#45069,#35938,#35939) ;
#30287=AXIS2_PLACEMENT_3D('',#45072,#35941,#35942) ;
#30288=AXIS2_PLACEMENT_3D('',#45073,#35943,#35944) ;
#30289=AXIS2_PLACEMENT_3D('',#45075,#35945,#35946) ;
#30290=AXIS2_PLACEMENT_3D('',#45078,#35948,#35949) ;
#30291=AXIS2_PLACEMENT_3D('',#45079,#35950,#35951) ;
#30292=AXIS2_PLACEMENT_3D('',#45081,#35952,#35953) ;
#30293=AXIS2_PLACEMENT_3D('',#45084,#35955,#35956) ;
#30294=AXIS2_PLACEMENT_3D('',#45085,#35957,#35958) ;
#30295=AXIS2_PLACEMENT_3D('',#45087,#35959,#35960) ;
#30296=AXIS2_PLACEMENT_3D('',#45090,#35962,#35963) ;
#30297=AXIS2_PLACEMENT_3D('',#45091,#35964,#35965) ;
#30298=AXIS2_PLACEMENT_3D('',#45096,#35967,#35968) ;
#30299=AXIS2_PLACEMENT_3D('',#45099,#35970,#35971) ;
#30300=AXIS2_PLACEMENT_3D('',#45100,#35972,#35973) ;
#30301=AXIS2_PLACEMENT_3D('',#45102,#35975,#35976) ;
#30302=AXIS2_PLACEMENT_3D('',#45108,#35979,#35980) ;
#30303=AXIS2_PLACEMENT_3D('',#45110,#35981,#35982) ;
#30304=AXIS2_PLACEMENT_3D('',#45112,#35983,#35984) ;
#30305=AXIS2_PLACEMENT_3D('',#45114,#35985,#35986) ;
#30306=AXIS2_PLACEMENT_3D('',#45115,#35987,#35988) ;
#30307=AXIS2_PLACEMENT_3D('',#45121,#35991,#35992) ;
#30308=AXIS2_PLACEMENT_3D('',#45125,#35994,#35995) ;
#30309=AXIS2_PLACEMENT_3D('',#45133,#35999,#36000) ;
#30310=AXIS2_PLACEMENT_3D('',#45135,#36002,#36003) ;
#30311=AXIS2_PLACEMENT_3D('',#45139,#36005,#36006) ;
#30312=AXIS2_PLACEMENT_3D('',#45140,#36007,#36008) ;
#30313=AXIS2_PLACEMENT_3D('',#45143,#36011,#36012) ;
#30314=AXIS2_PLACEMENT_3D('',#45166,#36024,#36025) ;
#30315=AXIS2_PLACEMENT_3D('',#45167,#36026,#36027) ;
#30316=AXIS2_PLACEMENT_3D('',#45171,#36029,#36030) ;
#30317=AXIS2_PLACEMENT_3D('',#45172,#36031,#36032) ;
#30318=AXIS2_PLACEMENT_3D('',#45175,#36035,#36036) ;
#30319=AXIS2_PLACEMENT_3D('',#45203,#36051,#36052) ;
#30320=AXIS2_PLACEMENT_3D('',#45204,#36053,#36054) ;
#30321=AXIS2_PLACEMENT_3D('',#45205,#36055,#36056) ;
#30322=AXIS2_PLACEMENT_3D('',#45206,#36057,#36058) ;
#30323=AXIS2_PLACEMENT_3D('',#45207,#36059,#36060) ;
#30324=AXIS2_PLACEMENT_3D('',#45209,#36061,#36062) ;
#30325=AXIS2_PLACEMENT_3D('',#45212,#36064,#36065) ;
#30326=AXIS2_PLACEMENT_3D('',#45213,#36066,#36067) ;
#30327=AXIS2_PLACEMENT_3D('',#45214,#36068,#36069) ;
#30328=AXIS2_PLACEMENT_3D('',#45216,#36070,#36071) ;
#30329=AXIS2_PLACEMENT_3D('',#45218,#36073,#36074) ;
#30330=AXIS2_PLACEMENT_3D('',#45219,#36075,#36076) ;
#30331=AXIS2_PLACEMENT_3D('',#45224,#36078,#36079) ;
#30332=AXIS2_PLACEMENT_3D('',#45227,#36081,#36082) ;
#30333=AXIS2_PLACEMENT_3D('',#45228,#36083,#36084) ;
#30334=AXIS2_PLACEMENT_3D('',#45233,#36086,#36087) ;
#30335=AXIS2_PLACEMENT_3D('',#45236,#36089,#36090) ;
#30336=AXIS2_PLACEMENT_3D('',#45237,#36091,#36092) ;
#30337=AXIS2_PLACEMENT_3D('',#45247,#36098,#36099) ;
#30338=AXIS2_PLACEMENT_3D('',#45251,#36102,#36103) ;
#30339=AXIS2_PLACEMENT_3D('',#45255,#36106,#36107) ;
#30340=AXIS2_PLACEMENT_3D('',#45265,#36113,#36114) ;
#30341=AXIS2_PLACEMENT_3D('',#45269,#36117,#36118) ;
#30342=AXIS2_PLACEMENT_3D('',#45273,#36121,#36122) ;
#30343=AXIS2_PLACEMENT_3D('',#45277,#36125,#36126) ;
#30344=AXIS2_PLACEMENT_3D('',#45281,#36129,#36130) ;
#30345=AXIS2_PLACEMENT_3D('',#45283,#36132,#36133) ;
#30346=AXIS2_PLACEMENT_3D('',#45287,#36136,#36137) ;
#30347=AXIS2_PLACEMENT_3D('',#45291,#36140,#36141) ;
#30348=AXIS2_PLACEMENT_3D('',#45293,#36143,#36144) ;
#30349=AXIS2_PLACEMENT_3D('',#45296,#36145,#36146) ;
#30350=AXIS2_PLACEMENT_3D('',#45297,#36147,#36148) ;
#30351=AXIS2_PLACEMENT_3D('',#45298,#36149,#36150) ;
#30352=AXIS2_PLACEMENT_3D('',#45300,#36151,#36152) ;
#30353=AXIS2_PLACEMENT_3D('',#45304,#36156,#36157) ;
#30354=AXIS2_PLACEMENT_3D('',#45306,#36158,#36159) ;
#30355=AXIS2_PLACEMENT_3D('',#45308,#36161,#36162) ;
#30356=AXIS2_PLACEMENT_3D('',#45310,#36163,#36164) ;
#30357=AXIS2_PLACEMENT_3D('',#45313,#36166,#36167) ;
#30358=AXIS2_PLACEMENT_3D('',#45314,#36168,#36169) ;
#30359=AXIS2_PLACEMENT_3D('',#45315,#36170,#36171) ;
#30360=AXIS2_PLACEMENT_3D('',#45316,#36172,#36173) ;
#30361=AXIS2_PLACEMENT_3D('',#45318,#36174,#36175) ;
#30362=AXIS2_PLACEMENT_3D('',#45321,#36177,#36178) ;
#30363=AXIS2_PLACEMENT_3D('',#45322,#36179,#36180) ;
#30364=AXIS2_PLACEMENT_3D('',#45323,#36181,#36182) ;
#30365=AXIS2_PLACEMENT_3D('',#45325,#36183,#36184) ;
#30366=AXIS2_PLACEMENT_3D('',#45328,#36186,#36187) ;
#30367=AXIS2_PLACEMENT_3D('',#45329,#36188,#36189) ;
#30368=AXIS2_PLACEMENT_3D('',#45330,#36190,#36191) ;
#30369=AXIS2_PLACEMENT_3D('',#45332,#36192,#36193) ;
#30370=AXIS2_PLACEMENT_3D('',#45335,#36195,#36196) ;
#30371=AXIS2_PLACEMENT_3D('',#45336,#36197,#36198) ;
#30372=AXIS2_PLACEMENT_3D('',#45337,#36199,#36200) ;
#30373=AXIS2_PLACEMENT_3D('',#45340,#36202,#36203) ;
#30374=AXIS2_PLACEMENT_3D('',#45341,#36204,#36205) ;
#30375=AXIS2_PLACEMENT_3D('',#45342,#36206,#36207) ;
#30376=AXIS2_PLACEMENT_3D('',#45348,#36211,#36212) ;
#30377=AXIS2_PLACEMENT_3D('',#45354,#36216,#36217) ;
#30378=AXIS2_PLACEMENT_3D('',#45356,#36219,#36220) ;
#30379=AXIS2_PLACEMENT_3D('',#45358,#36222,#36223) ;
#30380=AXIS2_PLACEMENT_3D('',#45365,#36228,#36229) ;
#30381=AXIS2_PLACEMENT_3D('',#45371,#36233,#36234) ;
#30382=AXIS2_PLACEMENT_3D('',#45377,#36238,#36239) ;
#30383=AXIS2_PLACEMENT_3D('',#45379,#36241,#36242) ;
#30384=AXIS2_PLACEMENT_3D('',#45381,#36244,#36245) ;
#30385=AXIS2_PLACEMENT_3D('',#45385,#36248,#36249) ;
#30386=AXIS2_PLACEMENT_3D('',#45389,#36252,#36253) ;
#30387=AXIS2_PLACEMENT_3D('',#45391,#36255,#36256) ;
#30388=AXIS2_PLACEMENT_3D('',#45392,#36257,#36258) ;
#30389=AXIS2_PLACEMENT_3D('',#45398,#36262,#36263) ;
#30390=AXIS2_PLACEMENT_3D('',#45404,#36267,#36268) ;
#30391=AXIS2_PLACEMENT_3D('',#45407,#36271,#36272) ;
#30392=AXIS2_PLACEMENT_3D('',#45408,#36273,#36274) ;
#30393=AXIS2_PLACEMENT_3D('',#45410,#36276,#36277) ;
#35934=DIRECTION('axis',(0.,0.,1.)) ;
#35935=DIRECTION('refdir',(1.,0.,0.)) ;
#35936=DIRECTION('center_axis',(0.,0.,1.)) ;
#35937=DIRECTION('ref_axis',(1.,0.,0.)) ;
#35938=DIRECTION('center_axis',(0.,0.,1.)) ;
#35939=DIRECTION('ref_axis',(1.,0.,0.)) ;
#35940=DIRECTION('',(0.,0.,1.)) ;
#35941=DIRECTION('center_axis',(0.,0.,-1.)) ;
#35942=DIRECTION('ref_axis',(1.,0.,0.)) ;
#35943=DIRECTION('center_axis',(0.,0.,1.)) ;
#35944=DIRECTION('ref_axis',(1.,0.,0.)) ;
#35945=DIRECTION('center_axis',(0.,0.,1.)) ;
#35946=DIRECTION('ref_axis',(1.,0.,0.)) ;
#35947=DIRECTION('',(0.,0.,1.)) ;
#35948=DIRECTION('center_axis',(0.,0.,-1.)) ;
#35949=DIRECTION('ref_axis',(1.,0.,0.)) ;
#35950=DIRECTION('center_axis',(0.,0.,1.)) ;
#35951=DIRECTION('ref_axis',(1.,0.,0.)) ;
#35952=DIRECTION('center_axis',(0.,0.,1.)) ;
#35953=DIRECTION('ref_axis',(1.,0.,0.)) ;
#35954=DIRECTION('',(0.,0.,1.)) ;
#35955=DIRECTION('center_axis',(0.,0.,-1.)) ;
#35956=DIRECTION('ref_axis',(1.,0.,0.)) ;
#35957=DIRECTION('center_axis',(0.,0.,1.)) ;
#35958=DIRECTION('ref_axis',(1.,0.,0.)) ;
#35959=DIRECTION('center_axis',(0.,0.,1.)) ;
#35960=DIRECTION('ref_axis',(1.,0.,0.)) ;
#35961=DIRECTION('',(0.,0.,1.)) ;
#35962=DIRECTION('center_axis',(0.,0.,-1.)) ;
#35963=DIRECTION('ref_axis',(1.,0.,0.)) ;
#35964=DIRECTION('center_axis',(0.,0.,1.)) ;
#35965=DIRECTION('ref_axis',(1.,0.,0.)) ;
#35966=DIRECTION('',(0.,0.,1.)) ;
#35967=DIRECTION('center_axis',(0.,0.,-1.)) ;
#35968=DIRECTION('ref_axis',(1.,0.,0.)) ;
#35969=DIRECTION('',(0.,0.,-1.)) ;
#35970=DIRECTION('center_axis',(0.,0.,-1.)) ;
#35971=DIRECTION('ref_axis',(1.,0.,0.)) ;
#35972=DIRECTION('center_axis',(0.,0.,-1.)) ;
#35973=DIRECTION('ref_axis',(-1.,0.,0.)) ;
#35974=DIRECTION('',(0.,1.,0.)) ;
#35975=DIRECTION('center_axis',(0.,0.,1.)) ;
#35976=DIRECTION('ref_axis',(1.,0.,0.)) ;
#35977=DIRECTION('',(0.,-1.,0.)) ;
#35978=DIRECTION('',(1.,0.,0.)) ;
#35979=DIRECTION('center_axis',(0.,0.,-1.)) ;
#35980=DIRECTION('ref_axis',(1.,0.,0.)) ;
#35981=DIRECTION('center_axis',(0.,0.,-1.)) ;
#35982=DIRECTION('ref_axis',(1.,0.,0.)) ;
#35983=DIRECTION('center_axis',(0.,0.,-1.)) ;
#35984=DIRECTION('ref_axis',(1.,0.,0.)) ;
#35985=DIRECTION('center_axis',(0.,0.,-1.)) ;
#35986=DIRECTION('ref_axis',(1.,0.,0.)) ;
#35987=DIRECTION('center_axis',(0.,0.,-1.)) ;
#35988=DIRECTION('ref_axis',(1.,0.,0.)) ;
#35989=DIRECTION('',(1.,0.,0.)) ;
#35990=DIRECTION('',(0.,1.,0.)) ;
#35991=DIRECTION('center_axis',(0.,0.,-1.)) ;
#35992=DIRECTION('ref_axis',(1.,0.,0.)) ;
#35993=DIRECTION('',(0.,1.,0.)) ;
#35994=DIRECTION('center_axis',(0.,0.,-1.)) ;
#35995=DIRECTION('ref_axis',(1.,0.,0.)) ;
#35996=DIRECTION('',(0.,1.,0.)) ;
#35997=DIRECTION('',(-1.,0.,0.)) ;
#35998=DIRECTION('',(0.,-1.,0.)) ;
#35999=DIRECTION('center_axis',(0.,0.,-1.)) ;
#36000=DIRECTION('ref_axis',(1.,0.,0.)) ;
#36001=DIRECTION('',(0.,-1.,0.)) ;
#36002=DIRECTION('center_axis',(0.,0.,-1.)) ;
#36003=DIRECTION('ref_axis',(-1.,0.,0.)) ;
#36004=DIRECTION('',(0.,1.,0.)) ;
#36005=DIRECTION('center_axis',(0.,0.,-1.)) ;
#36006=DIRECTION('ref_axis',(1.,0.,0.)) ;
#36007=DIRECTION('center_axis',(0.,0.,1.)) ;
#36008=DIRECTION('ref_axis',(1.,0.,0.)) ;
#36009=DIRECTION('',(0.,0.,-1.)) ;
#36010=DIRECTION('',(0.,0.,1.)) ;
#36011=DIRECTION('center_axis',(1.,0.,0.)) ;
#36012=DIRECTION('ref_axis',(0.,0.,-1.)) ;
#36013=DIRECTION('',(0.,0.,-1.)) ;
#36014=DIRECTION('',(0.,-1.,0.)) ;
#36015=DIRECTION('',(0.,0.,-1.)) ;
#36016=DIRECTION('',(0.,1.,0.)) ;
#36017=DIRECTION('',(0.,0.,-1.)) ;
#36018=DIRECTION('',(0.,1.,0.)) ;
#36019=DIRECTION('',(0.,0.,-1.)) ;
#36020=DIRECTION('',(0.,1.,0.)) ;
#36021=DIRECTION('',(0.,0.,-1.)) ;
#36022=DIRECTION('',(0.,-1.,0.)) ;
#36023=DIRECTION('',(0.,0.,-1.)) ;
#36024=DIRECTION('center_axis',(1.,0.,0.)) ;
#36025=DIRECTION('ref_axis',(0.,0.,-1.)) ;
#36026=DIRECTION('center_axis',(0.,0.,-1.)) ;
#36027=DIRECTION('ref_axis',(-1.,0.,0.)) ;
#36028=DIRECTION('',(0.,-1.,0.)) ;
#36029=DIRECTION('center_axis',(0.,0.,-1.)) ;
#36030=DIRECTION('ref_axis',(1.,0.,0.)) ;
#36031=DIRECTION('center_axis',(0.,0.,1.)) ;
#36032=DIRECTION('ref_axis',(-1.,1.22464679914735E-16,0.)) ;
#36033=DIRECTION('',(0.,0.,-1.)) ;
#36034=DIRECTION('',(0.,0.,1.)) ;
#36035=DIRECTION('center_axis',(-1.,0.,0.)) ;
#36036=DIRECTION('ref_axis',(0.,0.,1.)) ;
#36037=DIRECTION('',(0.,0.,-1.)) ;
#36038=DIRECTION('',(0.,1.,0.)) ;
#36039=DIRECTION('',(0.,0.,-1.)) ;
#36040=DIRECTION('',(0.,-1.,0.)) ;
#36041=DIRECTION('',(0.,0.,-1.)) ;
#36042=DIRECTION('',(0.,-1.,0.)) ;
#36043=DIRECTION('',(0.,0.,-1.)) ;
#36044=DIRECTION('',(0.,-1.,0.)) ;
#36045=DIRECTION('',(0.,0.,-1.)) ;
#36046=DIRECTION('',(0.,1.,0.)) ;
#36047=DIRECTION('',(0.,0.,-1.)) ;
#36048=DIRECTION('',(0.,0.,-1.)) ;
#36049=DIRECTION('',(0.,-1.,0.)) ;
#36050=DIRECTION('',(0.,0.,1.)) ;
#36051=DIRECTION('center_axis',(-1.,0.,0.)) ;
#36052=DIRECTION('ref_axis',(0.,0.,-1.)) ;
#36053=DIRECTION('center_axis',(0.,0.,-1.)) ;
#36054=DIRECTION('ref_axis',(-1.,0.,0.)) ;
#36055=DIRECTION('center_axis',(0.,0.,-1.)) ;
#36056=DIRECTION('ref_axis',(1.,0.,0.)) ;
#36057=DIRECTION('center_axis',(0.,0.,1.)) ;
#36058=DIRECTION('ref_axis',(-1.,1.22464679914735E-16,0.)) ;
#36059=DIRECTION('center_axis',(1.,0.,0.)) ;
#36060=DIRECTION('ref_axis',(0.,0.,-1.)) ;
#36061=DIRECTION('center_axis',(-1.,0.,0.)) ;
#36062=DIRECTION('ref_axis',(0.,0.,-1.)) ;
#36063=DIRECTION('',(1.,0.,0.)) ;
#36064=DIRECTION('center_axis',(-1.,0.,0.)) ;
#36065=DIRECTION('ref_axis',(0.,0.,-1.)) ;
#36066=DIRECTION('center_axis',(-1.,0.,0.)) ;
#36067=DIRECTION('ref_axis',(0.,0.,1.)) ;
#36068=DIRECTION('center_axis',(1.,0.,0.)) ;
#36069=DIRECTION('ref_axis',(0.,0.,-1.)) ;
#36070=DIRECTION('center_axis',(1.,0.,0.)) ;
#36071=DIRECTION('ref_axis',(0.,0.,-1.)) ;
#36072=DIRECTION('',(-1.,0.,0.)) ;
#36073=DIRECTION('center_axis',(1.,0.,0.)) ;
#36074=DIRECTION('ref_axis',(0.,0.,-1.)) ;
#36075=DIRECTION('center_axis',(1.,0.,0.)) ;
#36076=DIRECTION('ref_axis',(0.,-1.22464679914735E-16,1.)) ;
#36077=DIRECTION('',(1.,0.,0.)) ;
#36078=DIRECTION('center_axis',(1.,0.,0.)) ;
#36079=DIRECTION('ref_axis',(0.,0.,-1.)) ;
#36080=DIRECTION('',(-1.,0.,0.)) ;
#36081=DIRECTION('center_axis',(-1.,0.,0.)) ;
#36082=DIRECTION('ref_axis',(0.,0.,-1.)) ;
#36083=DIRECTION('center_axis',(1.,0.,0.)) ;
#36084=DIRECTION('ref_axis',(0.,-1.22464679914735E-16,1.)) ;
#36085=DIRECTION('',(1.,0.,0.)) ;
#36086=DIRECTION('center_axis',(1.,0.,0.)) ;
#36087=DIRECTION('ref_axis',(0.,0.,-1.)) ;
#36088=DIRECTION('',(-1.,0.,0.)) ;
#36089=DIRECTION('center_axis',(-1.,0.,0.)) ;
#36090=DIRECTION('ref_axis',(0.,0.,-1.)) ;
#36091=DIRECTION('center_axis',(1.,0.,0.)) ;
#36092=DIRECTION('ref_axis',(0.,0.,-1.)) ;
#36093=DIRECTION('',(0.,1.,0.)) ;
#36094=DIRECTION('',(0.,0.,-1.)) ;
#36095=DIRECTION('',(0.,-1.,0.)) ;
#36096=DIRECTION('',(0.,0.,-1.)) ;
#36097=DIRECTION('',(0.,1.,0.)) ;
#36098=DIRECTION('center_axis',(0.,0.,1.)) ;
#36099=DIRECTION('ref_axis',(1.,0.,0.)) ;
#36100=DIRECTION('',(0.,-1.,0.)) ;
#36101=DIRECTION('',(-1.,0.,0.)) ;
#36102=DIRECTION('center_axis',(0.,0.,1.)) ;
#36103=DIRECTION('ref_axis',(1.,0.,0.)) ;
#36104=DIRECTION('',(1.,0.,0.)) ;
#36105=DIRECTION('',(0.,-1.,0.)) ;
#36106=DIRECTION('center_axis',(1.,0.,0.)) ;
#36107=DIRECTION('ref_axis',(0.,0.,-1.)) ;
#36108=DIRECTION('',(0.,1.,0.)) ;
#36109=DIRECTION('',(0.,0.,-1.)) ;
#36110=DIRECTION('',(0.,-1.,0.)) ;
#36111=DIRECTION('',(0.,0.,-1.)) ;
#36112=DIRECTION('',(0.,1.,0.)) ;
#36113=DIRECTION('center_axis',(0.,0.,1.)) ;
#36114=DIRECTION('ref_axis',(1.,0.,0.)) ;
#36115=DIRECTION('',(0.,-1.,0.)) ;
#36116=DIRECTION('',(-1.,0.,0.)) ;
#36117=DIRECTION('center_axis',(0.,0.,1.)) ;
#36118=DIRECTION('ref_axis',(1.,0.,0.)) ;
#36119=DIRECTION('',(1.,0.,0.)) ;
#36120=DIRECTION('',(0.,-1.,0.)) ;
#36121=DIRECTION('center_axis',(0.,1.,0.)) ;
#36122=DIRECTION('ref_axis',(0.,0.,1.)) ;
#36123=DIRECTION('',(0.,0.,-1.)) ;
#36124=DIRECTION('',(1.,0.,0.)) ;
#36125=DIRECTION('center_axis',(0.,-1.,0.)) ;
#36126=DIRECTION('ref_axis',(0.,0.,-1.)) ;
#36127=DIRECTION('',(0.,0.,-1.)) ;
#36128=DIRECTION('',(-1.,0.,0.)) ;
#36129=DIRECTION('center_axis',(-1.,0.,0.)) ;
#36130=DIRECTION('ref_axis',(0.,0.,1.)) ;
#36131=DIRECTION('',(0.,1.,0.)) ;
#36132=DIRECTION('center_axis',(0.,1.,0.)) ;
#36133=DIRECTION('ref_axis',(0.,0.,1.)) ;
#36134=DIRECTION('',(0.,0.,-1.)) ;
#36135=DIRECTION('',(1.,0.,0.)) ;
#36136=DIRECTION('center_axis',(0.,-1.,0.)) ;
#36137=DIRECTION('ref_axis',(0.,0.,-1.)) ;
#36138=DIRECTION('',(0.,0.,-1.)) ;
#36139=DIRECTION('',(-1.,0.,0.)) ;
#36140=DIRECTION('center_axis',(-1.,0.,0.)) ;
#36141=DIRECTION('ref_axis',(0.,0.,1.)) ;
#36142=DIRECTION('',(0.,1.,0.)) ;
#36143=DIRECTION('center_axis',(0.,0.,1.)) ;
#36144=DIRECTION('ref_axis',(1.,0.,0.)) ;
#36145=DIRECTION('center_axis',(0.,0.,1.)) ;
#36146=DIRECTION('ref_axis',(1.,0.,0.)) ;
#36147=DIRECTION('center_axis',(0.,0.,1.)) ;
#36148=DIRECTION('ref_axis',(1.,0.,0.)) ;
#36149=DIRECTION('center_axis',(0.,0.,1.)) ;
#36150=DIRECTION('ref_axis',(1.,0.,0.)) ;
#36151=DIRECTION('center_axis',(0.,0.,1.)) ;
#36152=DIRECTION('ref_axis',(1.,0.,0.)) ;
#36153=DIRECTION('',(0.,0.,1.)) ;
#36154=DIRECTION('',(0.,0.,-1.)) ;
#36155=DIRECTION('',(0.,0.,1.)) ;
#36156=DIRECTION('center_axis',(0.,0.,1.)) ;
#36157=DIRECTION('ref_axis',(1.,0.,0.)) ;
#36158=DIRECTION('center_axis',(0.,0.,1.)) ;
#36159=DIRECTION('ref_axis',(1.,0.,0.)) ;
#36160=DIRECTION('',(0.,0.,-1.)) ;
#36161=DIRECTION('center_axis',(0.,0.,1.)) ;
#36162=DIRECTION('ref_axis',(1.,0.,0.)) ;
#36163=DIRECTION('center_axis',(0.,0.,-1.)) ;
#36164=DIRECTION('ref_axis',(1.,0.,0.)) ;
#36165=DIRECTION('',(0.,0.,1.)) ;
#36166=DIRECTION('center_axis',(0.,0.,-1.)) ;
#36167=DIRECTION('ref_axis',(1.,0.,0.)) ;
#36168=DIRECTION('center_axis',(0.,0.,-1.)) ;
#36169=DIRECTION('ref_axis',(-1.,0.,0.)) ;
#36170=DIRECTION('center_axis',(0.,0.,1.)) ;
#36171=DIRECTION('ref_axis',(1.,0.,0.)) ;
#36172=DIRECTION('center_axis',(0.,1.,0.)) ;
#36173=DIRECTION('ref_axis',(1.,0.,0.)) ;
#36174=DIRECTION('center_axis',(0.,1.,0.)) ;
#36175=DIRECTION('ref_axis',(1.,0.,0.)) ;
#36176=DIRECTION('',(0.,1.,0.)) ;
#36177=DIRECTION('center_axis',(0.,1.,0.)) ;
#36178=DIRECTION('ref_axis',(1.,0.,0.)) ;
#36179=DIRECTION('center_axis',(0.,1.,0.)) ;
#36180=DIRECTION('ref_axis',(1.,0.,0.)) ;
#36181=DIRECTION('center_axis',(0.,1.,0.)) ;
#36182=DIRECTION('ref_axis',(1.,0.,0.)) ;
#36183=DIRECTION('center_axis',(0.,1.,0.)) ;
#36184=DIRECTION('ref_axis',(1.,0.,0.)) ;
#36185=DIRECTION('',(0.,-1.,0.)) ;
#36186=DIRECTION('center_axis',(0.,-1.,0.)) ;
#36187=DIRECTION('ref_axis',(1.,0.,0.)) ;
#36188=DIRECTION('center_axis',(0.,-1.,0.)) ;
#36189=DIRECTION('ref_axis',(-1.,0.,0.)) ;
#36190=DIRECTION('center_axis',(1.,0.,0.)) ;
#36191=DIRECTION('ref_axis',(0.,0.,-1.)) ;
#36192=DIRECTION('center_axis',(1.,0.,0.)) ;
#36193=DIRECTION('ref_axis',(0.,0.,-1.)) ;
#36194=DIRECTION('',(1.,0.,0.)) ;
#36195=DIRECTION('center_axis',(1.,0.,0.)) ;
#36196=DIRECTION('ref_axis',(0.,0.,-1.)) ;
#36197=DIRECTION('center_axis',(1.,0.,0.)) ;
#36198=DIRECTION('ref_axis',(0.,0.,-1.)) ;
#36199=DIRECTION('center_axis',(1.,0.,0.)) ;
#36200=DIRECTION('ref_axis',(0.,0.,-1.)) ;
#36201=DIRECTION('',(-1.,0.,0.)) ;
#36202=DIRECTION('center_axis',(-1.,0.,0.)) ;
#36203=DIRECTION('ref_axis',(0.,0.,-1.)) ;
#36204=DIRECTION('center_axis',(-1.,0.,0.)) ;
#36205=DIRECTION('ref_axis',(0.,0.,1.)) ;
#36206=DIRECTION('center_axis',(0.,0.,1.)) ;
#36207=DIRECTION('ref_axis',(1.,0.,0.)) ;
#36208=DIRECTION('',(0.,1.,0.)) ;
#36209=DIRECTION('',(1.,0.,0.)) ;
#36210=DIRECTION('',(1.,0.,0.)) ;
#36211=DIRECTION('center_axis',(0.,0.,1.)) ;
#36212=DIRECTION('ref_axis',(1.,0.,0.)) ;
#36213=DIRECTION('',(0.,-1.,0.)) ;
#36214=DIRECTION('',(-1.,0.,0.)) ;
#36215=DIRECTION('',(-1.,0.,0.)) ;
#36216=DIRECTION('center_axis',(0.,1.,0.)) ;
#36217=DIRECTION('ref_axis',(0.,0.,1.)) ;
#36218=DIRECTION('',(0.,0.,-1.)) ;
#36219=DIRECTION('center_axis',(-1.,0.,0.)) ;
#36220=DIRECTION('ref_axis',(0.,0.,1.)) ;
#36221=DIRECTION('',(0.,0.,-1.)) ;
#36222=DIRECTION('center_axis',(0.,1.,0.)) ;
#36223=DIRECTION('ref_axis',(0.,0.,1.)) ;
#36224=DIRECTION('',(-1.,0.,0.)) ;
#36225=DIRECTION('',(-1.,0.,0.)) ;
#36226=DIRECTION('',(0.,0.,1.)) ;
#36227=DIRECTION('',(1.,0.,0.)) ;
#36228=DIRECTION('center_axis',(0.,0.,1.)) ;
#36229=DIRECTION('ref_axis',(1.,0.,0.)) ;
#36230=DIRECTION('',(0.,1.,0.)) ;
#36231=DIRECTION('',(-1.,0.,0.)) ;
#36232=DIRECTION('',(-1.,0.,0.)) ;
#36233=DIRECTION('center_axis',(0.,0.,1.)) ;
#36234=DIRECTION('ref_axis',(1.,0.,0.)) ;
#36235=DIRECTION('',(0.,-1.,0.)) ;
#36236=DIRECTION('',(1.,0.,0.)) ;
#36237=DIRECTION('',(1.,0.,0.)) ;
#36238=DIRECTION('center_axis',(0.,-1.,0.)) ;
#36239=DIRECTION('ref_axis',(0.,0.,-1.)) ;
#36240=DIRECTION('',(0.,0.,-1.)) ;
#36241=DIRECTION('center_axis',(-1.,0.,0.)) ;
#36242=DIRECTION('ref_axis',(0.,0.,1.)) ;
#36243=DIRECTION('',(0.,0.,1.)) ;
#36244=DIRECTION('center_axis',(0.,0.,1.)) ;
#36245=DIRECTION('ref_axis',(1.,0.,0.)) ;
#36246=DIRECTION('',(0.,-1.,0.)) ;
#36247=DIRECTION('',(1.,0.,0.)) ;
#36248=DIRECTION('center_axis',(0.,0.,1.)) ;
#36249=DIRECTION('ref_axis',(1.,0.,0.)) ;
#36250=DIRECTION('',(-1.,0.,0.)) ;
#36251=DIRECTION('',(0.,1.,0.)) ;
#36252=DIRECTION('center_axis',(0.,1.,0.)) ;
#36253=DIRECTION('ref_axis',(0.,0.,1.)) ;
#36254=DIRECTION('',(0.,0.,-1.)) ;
#36255=DIRECTION('center_axis',(1.,0.,0.)) ;
#36256=DIRECTION('ref_axis',(0.,0.,-1.)) ;
#36257=DIRECTION('center_axis',(0.,0.,1.)) ;
#36258=DIRECTION('ref_axis',(1.,0.,0.)) ;
#36259=DIRECTION('',(-1.,0.,0.)) ;
#36260=DIRECTION('',(0.,-1.,0.)) ;
#36261=DIRECTION('',(-1.,0.,0.)) ;
#36262=DIRECTION('center_axis',(0.,0.,1.)) ;
#36263=DIRECTION('ref_axis',(1.,0.,0.)) ;
#36264=DIRECTION('',(1.,0.,0.)) ;
#36265=DIRECTION('',(0.,1.,0.)) ;
#36266=DIRECTION('',(1.,0.,0.)) ;
#36267=DIRECTION('center_axis',(1.,0.,0.)) ;
#36268=DIRECTION('ref_axis',(0.,0.,-1.)) ;
#36269=DIRECTION('',(0.,0.,-1.)) ;
#36270=DIRECTION('',(0.,0.,-1.)) ;
#36271=DIRECTION('center_axis',(0.,-1.,0.)) ;
#36272=DIRECTION('ref_axis',(0.,0.,-1.)) ;
#36273=DIRECTION('center_axis',(0.,-1.,0.)) ;
#36274=DIRECTION('ref_axis',(0.,0.,-1.)) ;
#36275=DIRECTION('',(1.,0.,0.)) ;
#36276=DIRECTION('center_axis',(0.,0.,1.)) ;
#36277=DIRECTION('ref_axis',(1.,0.,0.)) ;
#45066=CARTESIAN_POINT('',(0.,0.,0.)) ;
#45067=CARTESIAN_POINT('Origin',(-8.5,-22.,31.5)) ;
#45068=CARTESIAN_POINT('',(-9.15,-22.,31.)) ;
#45069=CARTESIAN_POINT('Origin',(-8.5,-22.,31.)) ;
#45070=CARTESIAN_POINT('',(-9.15,-22.,32.)) ;
#45071=CARTESIAN_POINT('',(-9.15,-22.,31.5)) ;
#45072=CARTESIAN_POINT('Origin',(-8.5,-22.,32.)) ;
#45073=CARTESIAN_POINT('Origin',(-8.5,22.,31.5)) ;
#45074=CARTESIAN_POINT('',(-9.15,22.,31.)) ;
#45075=CARTESIAN_POINT('Origin',(-8.5,22.,31.)) ;
#45076=CARTESIAN_POINT('',(-9.15,22.,32.)) ;
#45077=CARTESIAN_POINT('',(-9.15,22.,31.5)) ;
#45078=CARTESIAN_POINT('Origin',(-8.5,22.,32.)) ;
#45079=CARTESIAN_POINT('Origin',(8.5,-22.,31.5)) ;
#45080=CARTESIAN_POINT('',(7.85,-22.,31.)) ;
#45081=CARTESIAN_POINT('Origin',(8.5,-22.,31.)) ;
#45082=CARTESIAN_POINT('',(7.85,-22.,32.)) ;
#45083=CARTESIAN_POINT('',(7.85,-22.,31.5)) ;
#45084=CARTESIAN_POINT('Origin',(8.5,-22.,32.)) ;
#45085=CARTESIAN_POINT('Origin',(8.5,22.,31.5)) ;
#45086=CARTESIAN_POINT('',(7.85,22.,31.)) ;
#45087=CARTESIAN_POINT('Origin',(8.5,22.,31.)) ;
#45088=CARTESIAN_POINT('',(7.85,22.,32.)) ;
#45089=CARTESIAN_POINT('',(7.85,22.,31.5)) ;
#45090=CARTESIAN_POINT('Origin',(8.5,22.,32.)) ;
#45091=CARTESIAN_POINT('Origin',(-11.,-10.,41.05)) ;
#45092=CARTESIAN_POINT('',(-11.,-9.575,40.)) ;
#45093=CARTESIAN_POINT('',(-11.,-9.575,42.)) ;
#45094=CARTESIAN_POINT('',(-11.,-9.575,41.05)) ;
#45095=CARTESIAN_POINT('',(-11.,-10.425,40.)) ;
#45096=CARTESIAN_POINT('Origin',(-11.,-10.,40.)) ;
#45097=CARTESIAN_POINT('',(-11.,-10.425,42.)) ;
#45098=CARTESIAN_POINT('',(-11.,-10.425,41.05)) ;
#45099=CARTESIAN_POINT('Origin',(-11.,-10.,42.)) ;
#45100=CARTESIAN_POINT('Origin',(-11.,-10.,40.)) ;
#45101=CARTESIAN_POINT('',(-11.,-5.,40.)) ;
#45102=CARTESIAN_POINT('Origin',(0.,0.,42.)) ;
#45103=CARTESIAN_POINT('',(-11.,-11.,42.)) ;
#45104=CARTESIAN_POINT('',(-11.,0.,42.)) ;
#45105=CARTESIAN_POINT('',(0.,-11.,42.)) ;
#45106=CARTESIAN_POINT('',(0.,-11.,42.)) ;
#45107=CARTESIAN_POINT('',(-2.5,-8.5,42.)) ;
#45108=CARTESIAN_POINT('Origin',(0.,-8.5,42.)) ;
#45109=CARTESIAN_POINT('',(-1.79965394597392,-6.76470588235294,42.)) ;
#45110=CARTESIAN_POINT('Origin',(0.,-8.5,42.)) ;
#45111=CARTESIAN_POINT('',(-7.,-8.57252759403147E-16,42.)) ;
#45112=CARTESIAN_POINT('Origin',(0.,0.,42.)) ;
#45113=CARTESIAN_POINT('',(1.79965394597392,-6.76470588235294,42.)) ;
#45114=CARTESIAN_POINT('Origin',(0.,0.,42.)) ;
#45115=CARTESIAN_POINT('Origin',(0.,-8.5,42.)) ;
#45116=CARTESIAN_POINT('',(11.,-11.,42.)) ;
#45117=CARTESIAN_POINT('',(0.,-11.,42.)) ;
#45118=CARTESIAN_POINT('',(11.,-10.425,42.)) ;
#45119=CARTESIAN_POINT('',(11.,0.,42.)) ;
#45120=CARTESIAN_POINT('',(11.,-9.575,42.)) ;
#45121=CARTESIAN_POINT('Origin',(11.,-10.,42.)) ;
#45122=CARTESIAN_POINT('',(11.,9.575,42.)) ;
#45123=CARTESIAN_POINT('',(11.,0.,42.)) ;
#45124=CARTESIAN_POINT('',(11.,10.425,42.)) ;
#45125=CARTESIAN_POINT('Origin',(11.,10.,42.)) ;
#45126=CARTESIAN_POINT('',(11.,11.,42.)) ;
#45127=CARTESIAN_POINT('',(11.,0.,42.)) ;
#45128=CARTESIAN_POINT('',(-11.,11.,42.)) ;
#45129=CARTESIAN_POINT('',(0.,11.,42.)) ;
#45130=CARTESIAN_POINT('',(-11.,10.425,42.)) ;
#45131=CARTESIAN_POINT('',(-11.,0.,42.)) ;
#45132=CARTESIAN_POINT('',(-11.,9.575,42.)) ;
#45133=CARTESIAN_POINT('Origin',(-11.,10.,42.)) ;
#45134=CARTESIAN_POINT('',(-11.,0.,42.)) ;
#45135=CARTESIAN_POINT('Origin',(-11.,10.,40.)) ;
#45136=CARTESIAN_POINT('',(-11.,9.575,40.)) ;
#45137=CARTESIAN_POINT('',(-11.,10.425,40.)) ;
#45138=CARTESIAN_POINT('',(-11.,5.,40.)) ;
#45139=CARTESIAN_POINT('Origin',(-11.,10.,40.)) ;
#45140=CARTESIAN_POINT('Origin',(-11.,10.,41.05)) ;
#45141=CARTESIAN_POINT('',(-11.,9.575,41.05)) ;
#45142=CARTESIAN_POINT('',(-11.,10.425,41.05)) ;
#45143=CARTESIAN_POINT('Origin',(-11.,0.,34.)) ;
#45144=CARTESIAN_POINT('',(-11.,11.,32.)) ;
#45145=CARTESIAN_POINT('',(-11.,11.,34.)) ;
#45146=CARTESIAN_POINT('',(-11.,25.,32.)) ;
#45147=CARTESIAN_POINT('',(-11.,18.,32.)) ;
#45148=CARTESIAN_POINT('',(-11.,25.,31.)) ;
#45149=CARTESIAN_POINT('',(-11.,25.,31.5)) ;
#45150=CARTESIAN_POINT('',(-11.,11.,31.)) ;
#45151=CARTESIAN_POINT('',(-11.,18.,31.)) ;
#45152=CARTESIAN_POINT('',(-11.,11.,26.)) ;
#45153=CARTESIAN_POINT('',(-11.,11.,34.)) ;
#45154=CARTESIAN_POINT('',(-11.,-11.,26.)) ;
#45155=CARTESIAN_POINT('',(-11.,0.,26.)) ;
#45156=CARTESIAN_POINT('',(-11.,-11.,31.)) ;
#45157=CARTESIAN_POINT('',(-11.,-11.,34.)) ;
#45158=CARTESIAN_POINT('',(-11.,-25.,31.)) ;
#45159=CARTESIAN_POINT('',(-11.,-18.,31.)) ;
#45160=CARTESIAN_POINT('',(-11.,-25.,32.)) ;
#45161=CARTESIAN_POINT('',(-11.,-25.,31.5)) ;
#45162=CARTESIAN_POINT('',(-11.,-11.,32.)) ;
#45163=CARTESIAN_POINT('',(-11.,-18.,32.)) ;
#45164=CARTESIAN_POINT('',(-11.,-11.,34.)) ;
#45165=CARTESIAN_POINT('',(-11.,-4.28626379701574E-16,37.5)) ;
#45166=CARTESIAN_POINT('Origin',(-11.,0.,34.)) ;
#45167=CARTESIAN_POINT('Origin',(11.,-10.,40.)) ;
#45168=CARTESIAN_POINT('',(11.,-9.575,40.)) ;
#45169=CARTESIAN_POINT('',(11.,-10.425,40.)) ;
#45170=CARTESIAN_POINT('',(11.,-5.,40.)) ;
#45171=CARTESIAN_POINT('Origin',(11.,-10.,40.)) ;
#45172=CARTESIAN_POINT('Origin',(11.,-10.,41.05)) ;
#45173=CARTESIAN_POINT('',(11.,-9.575,41.05)) ;
#45174=CARTESIAN_POINT('',(11.,-10.425,41.05)) ;
#45175=CARTESIAN_POINT('Origin',(11.,0.,34.)) ;
#45176=CARTESIAN_POINT('',(11.,-11.,32.)) ;
#45177=CARTESIAN_POINT('',(11.,-11.,34.)) ;
#45178=CARTESIAN_POINT('',(11.,-25.,32.)) ;
#45179=CARTESIAN_POINT('',(11.,-18.,32.)) ;
#45180=CARTESIAN_POINT('',(11.,-25.,31.)) ;
#45181=CARTESIAN_POINT('',(11.,-25.,31.5)) ;
#45182=CARTESIAN_POINT('',(11.,-11.,31.)) ;
#45183=CARTESIAN_POINT('',(11.,-18.,31.)) ;
#45184=CARTESIAN_POINT('',(11.,-11.,26.)) ;
#45185=CARTESIAN_POINT('',(11.,-11.,34.)) ;
#45186=CARTESIAN_POINT('',(11.,11.,26.)) ;
#45187=CARTESIAN_POINT('',(11.,0.,26.)) ;
#45188=CARTESIAN_POINT('',(11.,11.,31.)) ;
#45189=CARTESIAN_POINT('',(11.,11.,34.)) ;
#45190=CARTESIAN_POINT('',(11.,25.,31.)) ;
#45191=CARTESIAN_POINT('',(11.,18.,31.)) ;
#45192=CARTESIAN_POINT('',(11.,25.,32.)) ;
#45193=CARTESIAN_POINT('',(11.,25.,31.5)) ;
#45194=CARTESIAN_POINT('',(11.,11.,32.)) ;
#45195=CARTESIAN_POINT('',(11.,18.,32.)) ;
#45196=CARTESIAN_POINT('',(11.,11.,34.)) ;
#45197=CARTESIAN_POINT('',(11.,10.425,40.)) ;
#45198=CARTESIAN_POINT('',(11.,10.425,41.05)) ;
#45199=CARTESIAN_POINT('',(11.,9.575,40.)) ;
#45200=CARTESIAN_POINT('',(11.,5.,40.)) ;
#45201=CARTESIAN_POINT('',(11.,9.575,41.05)) ;
#45202=CARTESIAN_POINT('',(11.,7.,39.)) ;
#45203=CARTESIAN_POINT('Origin',(11.,7.,38.)) ;
#45204=CARTESIAN_POINT('Origin',(11.,10.,40.)) ;
#45205=CARTESIAN_POINT('Origin',(11.,10.,40.)) ;
#45206=CARTESIAN_POINT('Origin',(11.,10.,41.05)) ;
#45207=CARTESIAN_POINT('Origin',(10.95,7.,38.)) ;
#45208=CARTESIAN_POINT('',(10.,7.,38.5)) ;
#45209=CARTESIAN_POINT('Origin',(10.,7.,38.)) ;
#45210=CARTESIAN_POINT('',(11.8,7.,38.5)) ;
#45211=CARTESIAN_POINT('',(10.95,7.,38.5)) ;
#45212=CARTESIAN_POINT('Origin',(11.8,7.,38.)) ;
#45213=CARTESIAN_POINT('Origin',(10.,7.,38.)) ;
#45214=CARTESIAN_POINT('Origin',(11.4,7.,38.)) ;
#45215=CARTESIAN_POINT('',(11.8,7.,39.)) ;
#45216=CARTESIAN_POINT('Origin',(11.8,7.,38.)) ;
#45217=CARTESIAN_POINT('',(11.4,7.,39.)) ;
#45218=CARTESIAN_POINT('Origin',(11.8,7.,38.)) ;
#45219=CARTESIAN_POINT('Origin',(0.,0.,24.)) ;
#45220=CARTESIAN_POINT('',(9.5,-0.200997512422418,23.)) ;
#45221=CARTESIAN_POINT('',(10.5,-0.200997512422418,23.)) ;
#45222=CARTESIAN_POINT('',(0.,-0.200997512422418,23.)) ;
#45223=CARTESIAN_POINT('',(9.5,0.200997512422418,23.)) ;
#45224=CARTESIAN_POINT('Origin',(9.5,0.,24.)) ;
#45225=CARTESIAN_POINT('',(10.5,0.200997512422418,23.)) ;
#45226=CARTESIAN_POINT('',(0.,0.200997512422418,23.)) ;
#45227=CARTESIAN_POINT('Origin',(10.5,0.,24.)) ;
#45228=CARTESIAN_POINT('Origin',(0.,0.,24.)) ;
#45229=CARTESIAN_POINT('',(-10.5,-0.200997512422418,23.)) ;
#45230=CARTESIAN_POINT('',(-9.5,-0.200997512422418,23.)) ;
#45231=CARTESIAN_POINT('',(0.,-0.200997512422418,23.)) ;
#45232=CARTESIAN_POINT('',(-10.5,0.200997512422418,23.)) ;
#45233=CARTESIAN_POINT('Origin',(-10.5,0.,24.)) ;
#45234=CARTESIAN_POINT('',(-9.5,0.200997512422418,23.)) ;
#45235=CARTESIAN_POINT('',(0.,0.200997512422418,23.)) ;
#45236=CARTESIAN_POINT('Origin',(-9.5,0.,24.)) ;
#45237=CARTESIAN_POINT('Origin',(-10.5,0.,24.5)) ;
#45238=CARTESIAN_POINT('',(-10.5,-2.,23.)) ;
#45239=CARTESIAN_POINT('',(-10.5,0.,23.)) ;
#45240=CARTESIAN_POINT('',(-10.5,-2.,26.)) ;
#45241=CARTESIAN_POINT('',(-10.5,-2.,24.5)) ;
#45242=CARTESIAN_POINT('',(-10.5,2.,26.)) ;
#45243=CARTESIAN_POINT('',(-10.5,0.,26.)) ;
#45244=CARTESIAN_POINT('',(-10.5,2.,23.)) ;
#45245=CARTESIAN_POINT('',(-10.5,2.,24.5)) ;
#45246=CARTESIAN_POINT('',(-10.5,0.,23.)) ;
#45247=CARTESIAN_POINT('Origin',(-10.,0.,23.)) ;
#45248=CARTESIAN_POINT('',(-9.5,-2.,23.)) ;
#45249=CARTESIAN_POINT('',(-9.5,0.,23.)) ;
#45250=CARTESIAN_POINT('',(-10.,-2.,23.)) ;
#45251=CARTESIAN_POINT('Origin',(-10.,0.,23.)) ;
#45252=CARTESIAN_POINT('',(-9.5,2.,23.)) ;
#45253=CARTESIAN_POINT('',(-10.,2.,23.)) ;
#45254=CARTESIAN_POINT('',(-9.5,0.,23.)) ;
#45255=CARTESIAN_POINT('Origin',(9.5,0.,24.5)) ;
#45256=CARTESIAN_POINT('',(9.5,-2.,23.)) ;
#45257=CARTESIAN_POINT('',(9.5,0.,23.)) ;
#45258=CARTESIAN_POINT('',(9.5,-2.,26.)) ;
#45259=CARTESIAN_POINT('',(9.5,-2.,24.5)) ;
#45260=CARTESIAN_POINT('',(9.5,2.,26.)) ;
#45261=CARTESIAN_POINT('',(9.5,0.,26.)) ;
#45262=CARTESIAN_POINT('',(9.5,2.,23.)) ;
#45263=CARTESIAN_POINT('',(9.5,2.,24.5)) ;
#45264=CARTESIAN_POINT('',(9.5,0.,23.)) ;
#45265=CARTESIAN_POINT('Origin',(10.,0.,23.)) ;
#45266=CARTESIAN_POINT('',(10.5,-2.,23.)) ;
#45267=CARTESIAN_POINT('',(10.5,0.,23.)) ;
#45268=CARTESIAN_POINT('',(10.,-2.,23.)) ;
#45269=CARTESIAN_POINT('Origin',(10.,0.,23.)) ;
#45270=CARTESIAN_POINT('',(10.5,2.,23.)) ;
#45271=CARTESIAN_POINT('',(10.,2.,23.)) ;
#45272=CARTESIAN_POINT('',(10.5,0.,23.)) ;
#45273=CARTESIAN_POINT('Origin',(-10.,-2.,24.5)) ;
#45274=CARTESIAN_POINT('',(-9.5,-2.,26.)) ;
#45275=CARTESIAN_POINT('',(-9.5,-2.,24.5)) ;
#45276=CARTESIAN_POINT('',(-5.,-2.,26.)) ;
#45277=CARTESIAN_POINT('Origin',(-10.,2.,24.5)) ;
#45278=CARTESIAN_POINT('',(-9.5,2.,26.)) ;
#45279=CARTESIAN_POINT('',(-9.5,2.,24.5)) ;
#45280=CARTESIAN_POINT('',(-5.,2.,26.)) ;
#45281=CARTESIAN_POINT('Origin',(-9.5,0.,24.5)) ;
#45282=CARTESIAN_POINT('',(-9.5,0.,26.)) ;
#45283=CARTESIAN_POINT('Origin',(10.,-2.,24.5)) ;
#45284=CARTESIAN_POINT('',(10.5,-2.,26.)) ;
#45285=CARTESIAN_POINT('',(10.5,-2.,24.5)) ;
#45286=CARTESIAN_POINT('',(5.,-2.,26.)) ;
#45287=CARTESIAN_POINT('Origin',(10.,2.,24.5)) ;
#45288=CARTESIAN_POINT('',(10.5,2.,26.)) ;
#45289=CARTESIAN_POINT('',(10.5,2.,24.5)) ;
#45290=CARTESIAN_POINT('',(5.,2.,26.)) ;
#45291=CARTESIAN_POINT('Origin',(10.5,0.,24.5)) ;
#45292=CARTESIAN_POINT('',(10.5,0.,26.)) ;
#45293=CARTESIAN_POINT('Origin',(0.,0.,42.1)) ;
#45294=CARTESIAN_POINT('',(1.79965394597392,-6.76470588235294,42.1)) ;
#45295=CARTESIAN_POINT('',(-1.79965394597392,-6.76470588235294,42.1)) ;
#45296=CARTESIAN_POINT('Origin',(0.,-8.5,42.1)) ;
#45297=CARTESIAN_POINT('Origin',(0.,0.,42.1)) ;
#45298=CARTESIAN_POINT('Origin',(0.,0.,34.)) ;
#45299=CARTESIAN_POINT('',(-7.,-8.57252759403147E-16,26.)) ;
#45300=CARTESIAN_POINT('Origin',(0.,0.,26.)) ;
#45301=CARTESIAN_POINT('',(-7.,-8.57252759403147E-16,34.)) ;
#45302=CARTESIAN_POINT('',(-1.79965394597392,-6.76470588235294,34.)) ;
#45303=CARTESIAN_POINT('',(1.79965394597392,-6.76470588235294,34.)) ;
#45304=CARTESIAN_POINT('Origin',(0.,-8.5,43.)) ;
#45305=CARTESIAN_POINT('',(-2.5,-8.5,44.)) ;
#45306=CARTESIAN_POINT('Origin',(0.,-8.5,44.)) ;
#45307=CARTESIAN_POINT('',(-2.5,-8.5,43.)) ;
#45308=CARTESIAN_POINT('Origin',(0.,-8.5,42.05)) ;
#45309=CARTESIAN_POINT('',(-1.02,-8.5,40.)) ;
#45310=CARTESIAN_POINT('Origin',(0.,-8.5,40.)) ;
#45311=CARTESIAN_POINT('',(-1.02,-8.5,44.)) ;
#45312=CARTESIAN_POINT('',(-1.02,-8.5,42.05)) ;
#45313=CARTESIAN_POINT('Origin',(0.,-8.5,44.)) ;
#45314=CARTESIAN_POINT('Origin',(0.,-8.5,40.)) ;
#45315=CARTESIAN_POINT('Origin',(0.,-8.5,44.)) ;
#45316=CARTESIAN_POINT('Origin',(0.,-11.55,37.)) ;
#45317=CARTESIAN_POINT('',(-1.51,-13.,37.)) ;
#45318=CARTESIAN_POINT('Origin',(0.,-13.,37.)) ;
#45319=CARTESIAN_POINT('',(-1.51,-10.,37.)) ;
#45320=CARTESIAN_POINT('',(-1.51,-11.55,37.)) ;
#45321=CARTESIAN_POINT('Origin',(0.,-10.,37.)) ;
#45322=CARTESIAN_POINT('Origin',(0.,-10.,37.)) ;
#45323=CARTESIAN_POINT('Origin',(0.,-12.,37.)) ;
#45324=CARTESIAN_POINT('',(-3.,-11.,37.)) ;
#45325=CARTESIAN_POINT('Origin',(0.,-11.,37.)) ;
#45326=CARTESIAN_POINT('',(-3.,-13.,37.)) ;
#45327=CARTESIAN_POINT('',(-3.,-12.,37.)) ;
#45328=CARTESIAN_POINT('Origin',(0.,-13.,37.)) ;
#45329=CARTESIAN_POINT('Origin',(0.,-13.,37.)) ;
#45330=CARTESIAN_POINT('Origin',(-12.05,0.,34.)) ;
#45331=CARTESIAN_POINT('',(-14.,-2.16762483449082E-16,35.77)) ;
#45332=CARTESIAN_POINT('Origin',(-14.,0.,34.)) ;
#45333=CARTESIAN_POINT('',(-10.,-2.16762483449082E-16,35.77)) ;
#45334=CARTESIAN_POINT('',(-12.05,-2.16762483449082E-16,35.77)) ;
#45335=CARTESIAN_POINT('Origin',(-10.,0.,34.)) ;
#45336=CARTESIAN_POINT('Origin',(-10.,0.,34.)) ;
#45337=CARTESIAN_POINT('Origin',(-12.5,0.,34.)) ;
#45338=CARTESIAN_POINT('',(-14.,-4.28626379701574E-16,37.5)) ;
#45339=CARTESIAN_POINT('',(-12.5,-4.28626379701574E-16,37.5)) ;
#45340=CARTESIAN_POINT('Origin',(-14.,0.,34.)) ;
#45341=CARTESIAN_POINT('Origin',(-14.,0.,34.)) ;
#45342=CARTESIAN_POINT('Origin',(-8.5,-18.,32.)) ;
#45343=CARTESIAN_POINT('',(-6.,-25.,32.)) ;
#45344=CARTESIAN_POINT('',(-6.,-11.,32.)) ;
#45345=CARTESIAN_POINT('',(-6.,-18.,32.)) ;
#45346=CARTESIAN_POINT('',(-4.25,-11.,32.)) ;
#45347=CARTESIAN_POINT('',(-8.5,-25.,32.)) ;
#45348=CARTESIAN_POINT('Origin',(-8.5,-18.,31.)) ;
#45349=CARTESIAN_POINT('',(-6.,-11.,31.)) ;
#45350=CARTESIAN_POINT('',(-6.,-25.,31.)) ;
#45351=CARTESIAN_POINT('',(-6.,-18.,31.)) ;
#45352=CARTESIAN_POINT('',(-8.5,-25.,31.)) ;
#45353=CARTESIAN_POINT('',(-4.25,-11.,31.)) ;
#45354=CARTESIAN_POINT('Origin',(-8.5,-25.,31.5)) ;
#45355=CARTESIAN_POINT('',(-6.,-25.,31.5)) ;
#45356=CARTESIAN_POINT('Origin',(-6.,-18.,31.5)) ;
#45357=CARTESIAN_POINT('',(-6.,-11.,32.75)) ;
#45358=CARTESIAN_POINT('Origin',(0.,-11.,34.)) ;
#45359=CARTESIAN_POINT('',(0.,-11.,26.)) ;
#45360=CARTESIAN_POINT('',(6.,-11.,31.)) ;
#45361=CARTESIAN_POINT('',(4.25,-11.,31.)) ;
#45362=CARTESIAN_POINT('',(6.,-11.,32.)) ;
#45363=CARTESIAN_POINT('',(6.,-11.,32.75)) ;
#45364=CARTESIAN_POINT('',(4.25,-11.,32.)) ;
#45365=CARTESIAN_POINT('Origin',(-8.5,18.,32.)) ;
#45366=CARTESIAN_POINT('',(-6.,11.,32.)) ;
#45367=CARTESIAN_POINT('',(-6.,25.,32.)) ;
#45368=CARTESIAN_POINT('',(-6.,18.,32.)) ;
#45369=CARTESIAN_POINT('',(-8.5,25.,32.)) ;
#45370=CARTESIAN_POINT('',(-4.25,11.,32.)) ;
#45371=CARTESIAN_POINT('Origin',(-8.5,18.,31.)) ;
#45372=CARTESIAN_POINT('',(-6.,25.,31.)) ;
#45373=CARTESIAN_POINT('',(-6.,11.,31.)) ;
#45374=CARTESIAN_POINT('',(-6.,18.,31.)) ;
#45375=CARTESIAN_POINT('',(-4.25,11.,31.)) ;
#45376=CARTESIAN_POINT('',(-8.5,25.,31.)) ;
#45377=CARTESIAN_POINT('Origin',(-8.5,25.,31.5)) ;
#45378=CARTESIAN_POINT('',(-6.,25.,31.5)) ;
#45379=CARTESIAN_POINT('Origin',(-6.,18.,31.5)) ;
#45380=CARTESIAN_POINT('',(-6.,11.,32.75)) ;
#45381=CARTESIAN_POINT('Origin',(8.5,-18.,32.)) ;
#45382=CARTESIAN_POINT('',(6.,-25.,32.)) ;
#45383=CARTESIAN_POINT('',(6.,-18.,32.)) ;
#45384=CARTESIAN_POINT('',(8.5,-25.,32.)) ;
#45385=CARTESIAN_POINT('Origin',(8.5,-18.,31.)) ;
#45386=CARTESIAN_POINT('',(6.,-25.,31.)) ;
#45387=CARTESIAN_POINT('',(8.5,-25.,31.)) ;
#45388=CARTESIAN_POINT('',(6.,-18.,31.)) ;
#45389=CARTESIAN_POINT('Origin',(8.5,-25.,31.5)) ;
#45390=CARTESIAN_POINT('',(6.,-25.,31.5)) ;
#45391=CARTESIAN_POINT('Origin',(6.,-18.,31.5)) ;
#45392=CARTESIAN_POINT('Origin',(8.5,18.,32.)) ;
#45393=CARTESIAN_POINT('',(6.,25.,32.)) ;
#45394=CARTESIAN_POINT('',(8.5,25.,32.)) ;
#45395=CARTESIAN_POINT('',(6.,11.,32.)) ;
#45396=CARTESIAN_POINT('',(6.,18.,32.)) ;
#45397=CARTESIAN_POINT('',(4.25,11.,32.)) ;
#45398=CARTESIAN_POINT('Origin',(8.5,18.,31.)) ;
#45399=CARTESIAN_POINT('',(6.,11.,31.)) ;
#45400=CARTESIAN_POINT('',(4.25,11.,31.)) ;
#45401=CARTESIAN_POINT('',(6.,25.,31.)) ;
#45402=CARTESIAN_POINT('',(6.,18.,31.)) ;
#45403=CARTESIAN_POINT('',(8.5,25.,31.)) ;
#45404=CARTESIAN_POINT('Origin',(6.,18.,31.5)) ;
#45405=CARTESIAN_POINT('',(6.,25.,31.5)) ;
#45406=CARTESIAN_POINT('',(6.,11.,32.75)) ;
#45407=CARTESIAN_POINT('Origin',(8.5,25.,31.5)) ;
#45408=CARTESIAN_POINT('Origin',(0.,11.,34.)) ;
#45409=CARTESIAN_POINT('',(0.,11.,26.)) ;
#45410=CARTESIAN_POINT('Origin',(0.,0.,26.)) ;
#50348=UNCERTAINTY_MEASURE_WITH_UNIT(LENGTH_MEASURE(0.001),#50441,
'DISTANCE_ACCURACY_VALUE',
'Maximum model space distance between geometric entities at asserted c
onnectivities') ;
#50387=UNCERTAINTY_MEASURE_WITH_UNIT(LENGTH_MEASURE(0.001),#50441,
'DISTANCE_ACCURACY_VALUE',
'Maximum model space distance between geometric entities at asserted c
onnectivities') ;
#50401=(
GEOMETRIC_REPRESENTATION_CONTEXT(3)
GLOBAL_UNCERTAINTY_ASSIGNED_CONTEXT((#50348))
GLOBAL_UNIT_ASSIGNED_CONTEXT((#50441,#50443,#50444))
REPRESENTATION_CONTEXT('','3D')
) ;
#50440=(
GEOMETRIC_REPRESENTATION_CONTEXT(3)
GLOBAL_UNCERTAINTY_ASSIGNED_CONTEXT((#50387))
GLOBAL_UNIT_ASSIGNED_CONTEXT((#50441,#50443,#50444))
REPRESENTATION_CONTEXT('','3D')
) ;
#50441=(
LENGTH_UNIT()
NAMED_UNIT(*)
SI_UNIT(.CENTI.,.METRE.)
) ;
#50443=(
NAMED_UNIT(*)
PLANE_ANGLE_UNIT()
SI_UNIT($,.RADIAN.)
) ;
#50444=(
NAMED_UNIT(*)
SI_UNIT($,.STERADIAN.)
SOLID_ANGLE_UNIT()
) ;
#50458=SHAPE_DEFINITION_REPRESENTATION(#50524,#50632) ;
#50524=PRODUCT_DEFINITION_SHAPE('',$,#50685) ;
#50632=SHAPE_REPRESENTATION('',(#30284),#50401) ;
#50671=PRODUCT_DEFINITION_CONTEXT('part definition',#50829,'design') ;
#50685=PRODUCT_DEFINITION('GEARBOX_OSCILLATION_HOUSING',
'GEARBOX_OSCILLATION_HOUSING',#50737,#50671) ;
#50737=PRODUCT_DEFINITION_FORMATION('',$,#50844) ;
#50829=APPLICATION_CONTEXT(
'Core Data for Automotive Mechanical Design Process') ;
#50830=PRODUCT_CONTEXT('part definition',#50829,'mechanical') ;
#50844=PRODUCT('GEARBOX_OSCILLATION_HOUSING','GEARBOX_OSCILLATION_HOUSING',
$,(#50830)) ;
#50886=PRESENTATION_STYLE_ASSIGNMENT((#50893)) ;
#50893=SURFACE_STYLE_USAGE(.BOTH.,#50900) ;
#50900=SURFACE_SIDE_STYLE('',(#50907)) ;
#50907=SURFACE_STYLE_FILL_AREA(#50914) ;
#50914=FILL_AREA_STYLE('Aluminum - Satin',(#50921)) ;
#50921=FILL_AREA_STYLE_COLOUR('Aluminum - Satin',#50928) ;
#50928=COLOUR_RGB('Aluminum - Satin', 0.09019608, 0.27058824, 0.51372549) ;
ENDSEC;
END-ISO-10303-21;
